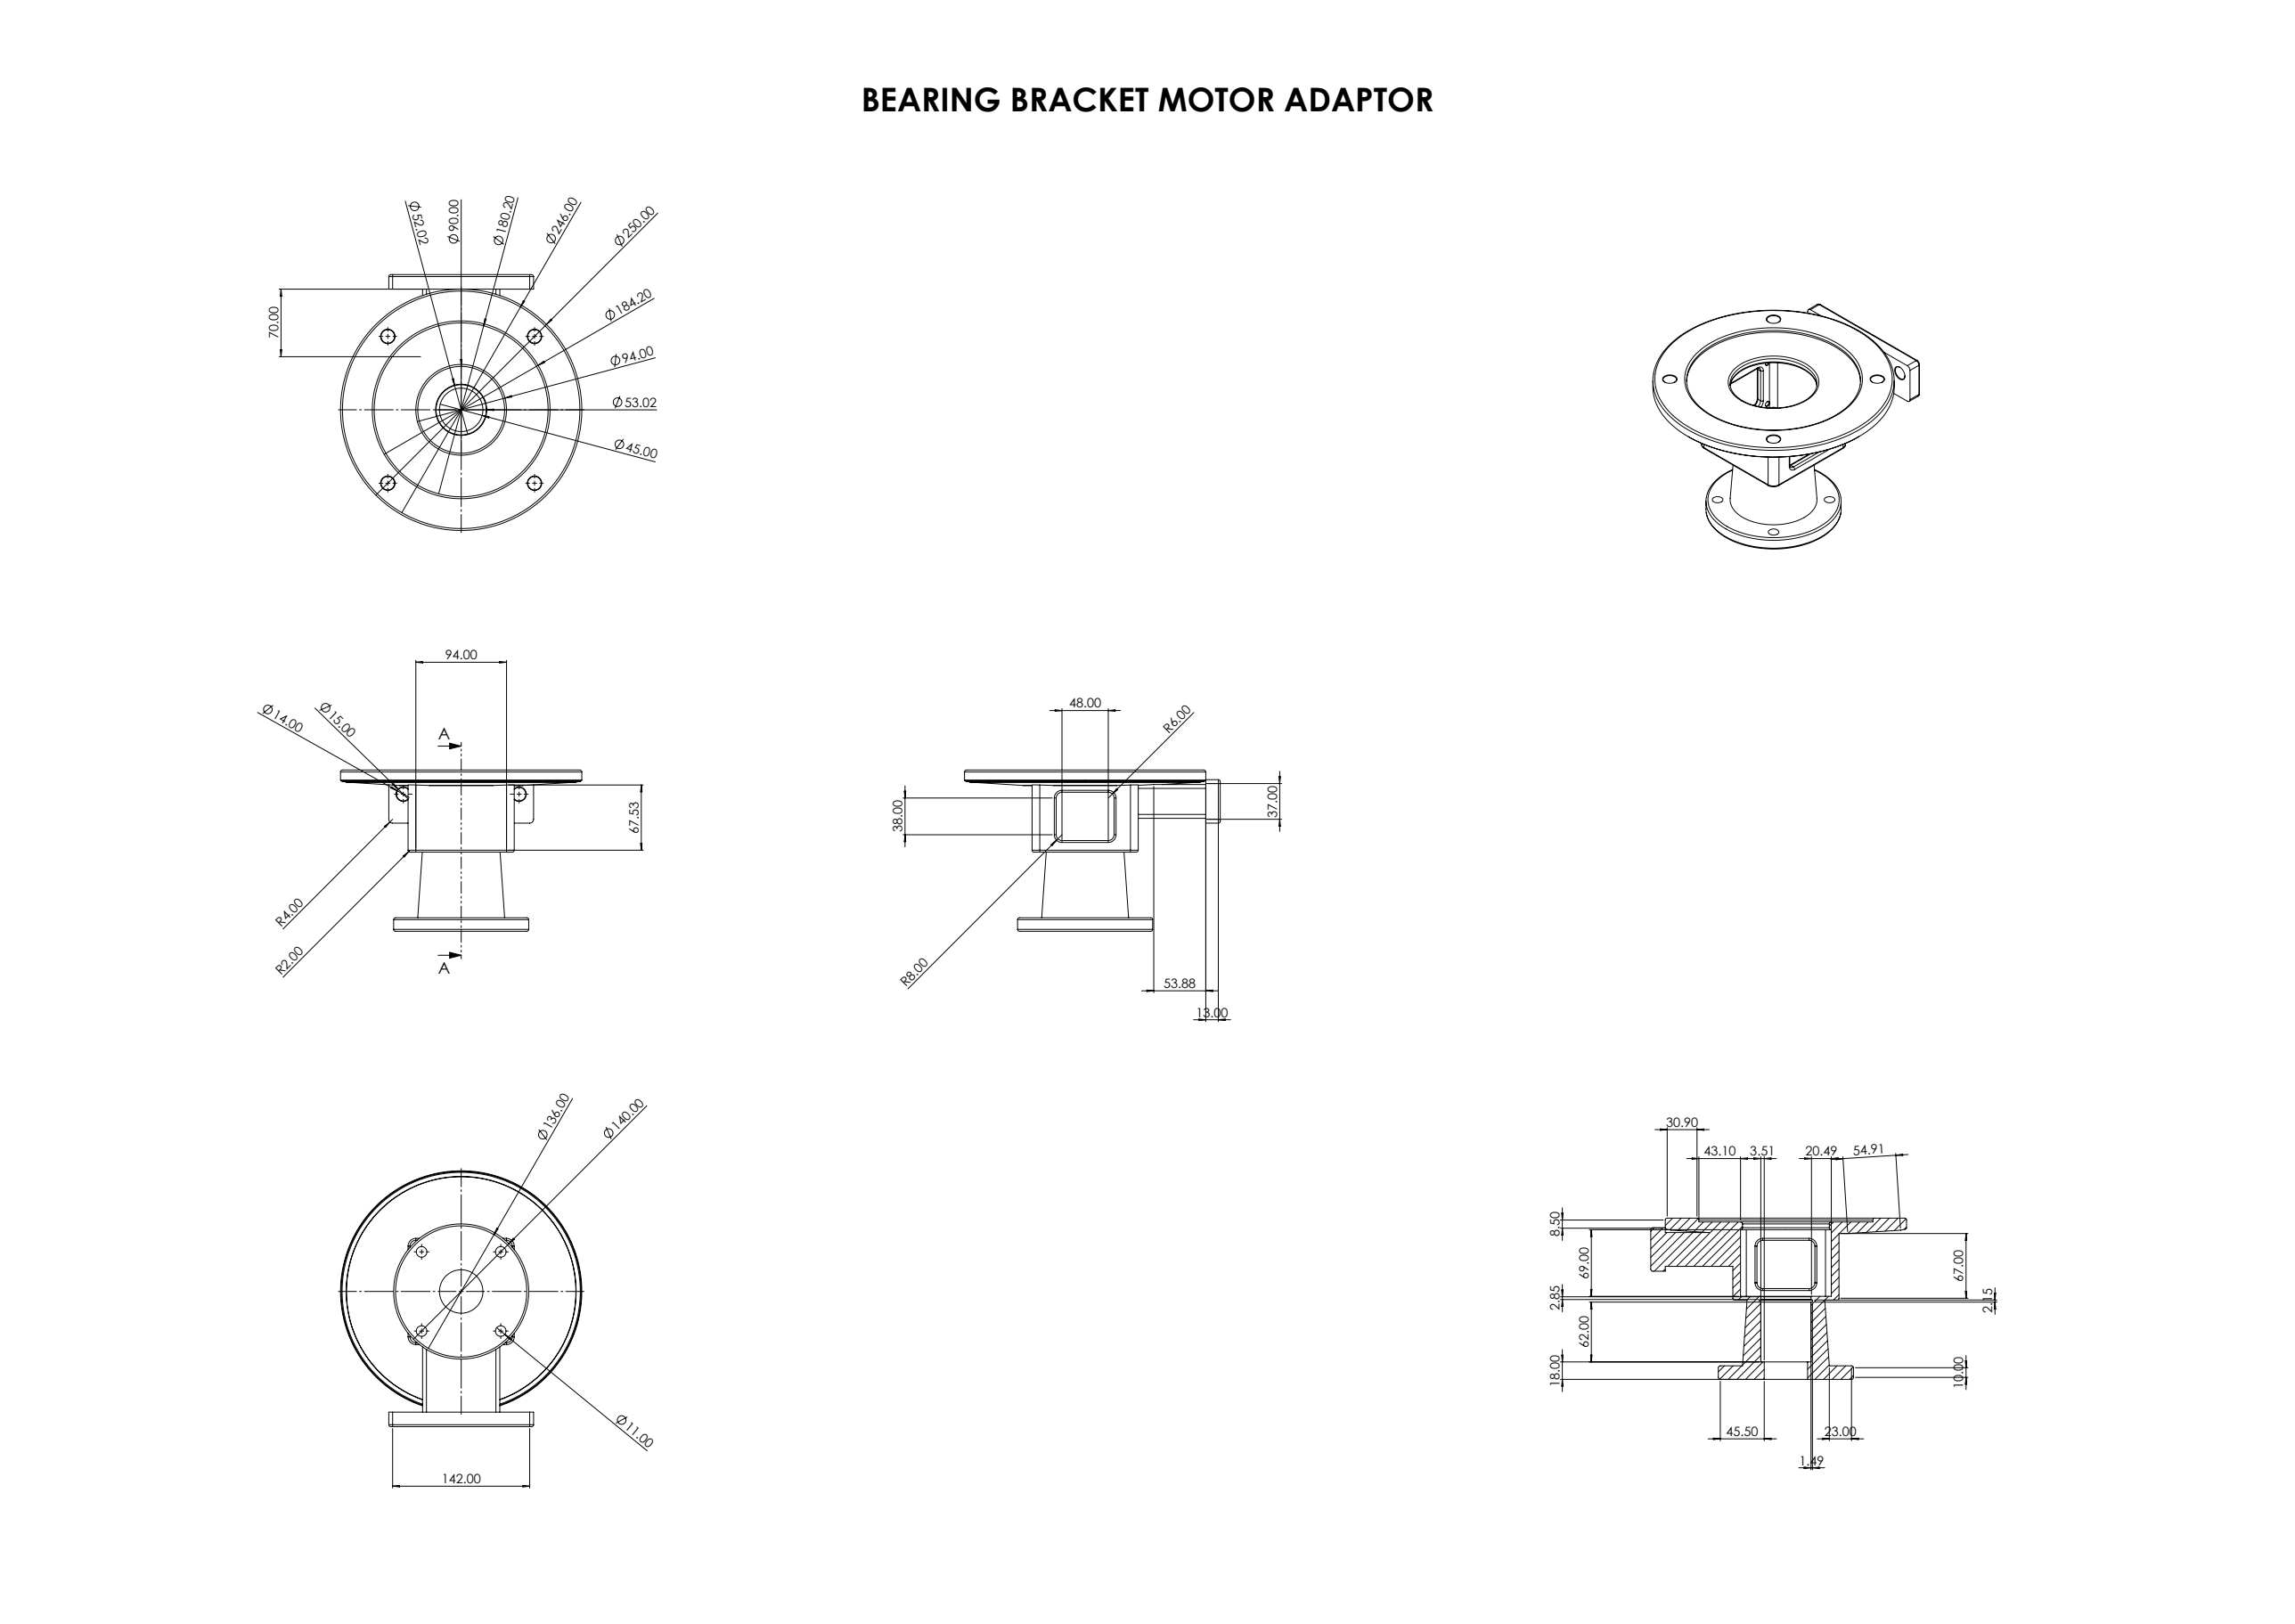
ISO-10303-21;
HEADER;
/* Generated by software containing ST-Developer
 * from STEP Tools, Inc. (www.steptools.com) 
 */

FILE_DESCRIPTION(
/* description */ (''),
/* implementation_level */ '2;1');

FILE_NAME(
/* name */ '03_Bearing_Bracket_Motor_Adaptor.step',
/* time_stamp */ '2026-10-26T04:15:57-07:00',
/* author */ (''),
/* organization */ (''),
/* preprocessor_version */ 'ST-DEVELOPER v20.2',
/* originating_system */ 'Autodesk Translation Framework v15.15.0.0',
/* authorisation */ '');

FILE_SCHEMA (('AUTOMOTIVE_DESIGN { 1 0 10303 214 3 1 1 }'));
ENDSEC;

DATA;
#10=MECHANICAL_DESIGN_GEOMETRIC_PRESENTATION_REPRESENTATION('',(#454),#55737);
#155=(
BOUNDED_CURVE()
B_SPLINE_CURVE(2,(#41789,#41790,#41791),.UNSPECIFIED.,.F.,.F.)
B_SPLINE_CURVE_WITH_KNOTS((3,3),(0.,1.18679419303782),.UNSPECIFIED.)
CURVE()
GEOMETRIC_REPRESENTATION_ITEM()
RATIONAL_B_SPLINE_CURVE((1.,1.03980835236638,1.06956749269866))
REPRESENTATION_ITEM('')
);
#156=(
BOUNDED_CURVE()
B_SPLINE_CURVE(2,(#41805,#41806,#41807),.UNSPECIFIED.,.F.,.F.)
B_SPLINE_CURVE_WITH_KNOTS((3,3),(8.21579802265979,9.40259221569659),
 .UNSPECIFIED.)
CURVE()
GEOMETRIC_REPRESENTATION_ITEM()
RATIONAL_B_SPLINE_CURVE((1.06956749269861,1.03980835236634,1.))
REPRESENTATION_ITEM('')
);
#157=(
BOUNDED_CURVE()
B_SPLINE_CURVE(2,(#41985,#41986,#41987),.UNSPECIFIED.,.F.,.F.)
B_SPLINE_CURVE_WITH_KNOTS((3,3),(0.,0.694054630120424),.UNSPECIFIED.)
CURVE()
GEOMETRIC_REPRESENTATION_ITEM()
RATIONAL_B_SPLINE_CURVE((1.,1.02328050763935,1.04312410261717))
REPRESENTATION_ITEM('')
);
#158=(
BOUNDED_CURVE()
B_SPLINE_CURVE(2,(#42011,#42012,#42013),.UNSPECIFIED.,.F.,.F.)
B_SPLINE_CURVE_WITH_KNOTS((3,3),(8.21579802265979,9.40259221569658),
 .UNSPECIFIED.)
CURVE()
GEOMETRIC_REPRESENTATION_ITEM()
RATIONAL_B_SPLINE_CURVE((1.06956749269861,1.03980835236634,1.))
REPRESENTATION_ITEM('')
);
#159=(
BOUNDED_CURVE()
B_SPLINE_CURVE(2,(#42017,#42018,#42019),.UNSPECIFIED.,.F.,.F.)
B_SPLINE_CURVE_WITH_KNOTS((3,3),(0.,1.18679419303782),.UNSPECIFIED.)
CURVE()
GEOMETRIC_REPRESENTATION_ITEM()
RATIONAL_B_SPLINE_CURVE((1.,1.03980835236638,1.06956749269866))
REPRESENTATION_ITEM('')
);
#160=(
BOUNDED_CURVE()
B_SPLINE_CURVE(2,(#42032,#42033,#42034),.UNSPECIFIED.,.F.,.F.)
B_SPLINE_CURVE_WITH_KNOTS((3,3),(8.21579802265979,9.40259221569659),
 .UNSPECIFIED.)
CURVE()
GEOMETRIC_REPRESENTATION_ITEM()
RATIONAL_B_SPLINE_CURVE((1.06956749269861,1.03980835236634,1.))
REPRESENTATION_ITEM('')
);
#161=(
BOUNDED_CURVE()
B_SPLINE_CURVE(2,(#42038,#42039,#42040),.UNSPECIFIED.,.F.,.F.)
B_SPLINE_CURVE_WITH_KNOTS((3,3),(0.,1.18679419303782),.UNSPECIFIED.)
CURVE()
GEOMETRIC_REPRESENTATION_ITEM()
RATIONAL_B_SPLINE_CURVE((1.,1.03980835236638,1.06956749269866))
REPRESENTATION_ITEM('')
);
#162=(
BOUNDED_CURVE()
B_SPLINE_CURVE(2,(#42053,#42054,#42055),.UNSPECIFIED.,.F.,.F.)
B_SPLINE_CURVE_WITH_KNOTS((3,3),(8.70853758557616,9.40259221569658),
 .UNSPECIFIED.)
CURVE()
GEOMETRIC_REPRESENTATION_ITEM()
RATIONAL_B_SPLINE_CURVE((1.04312410261717,1.02328050763935,1.))
REPRESENTATION_ITEM('')
);
#341=CONICAL_SURFACE('',#27990,26.26,0.785398163397439);
#342=CONICAL_SURFACE('',#28000,26.26,0.785398163397439);
#343=CONICAL_SURFACE('',#28004,7.25,0.785398163397439);
#344=CONICAL_SURFACE('',#28019,7.25,0.785398163397439);
#345=CONICAL_SURFACE('',#28023,2.8,0.785398163397448);
#346=CONICAL_SURFACE('',#28036,2.8,0.785398163397448);
#347=CONICAL_SURFACE('',#28043,2.8,0.785398163397448);
#348=CONICAL_SURFACE('',#28047,2.8,0.785398163397448);
#349=CONICAL_SURFACE('',#28052,2.8,0.785398163397448);
#350=CONICAL_SURFACE('',#28062,2.8,0.785398163397448);
#351=CONICAL_SURFACE('',#28063,2.8,0.785398163397448);
#352=CONICAL_SURFACE('',#28064,2.8,0.785398163397448);
#353=CONICAL_SURFACE('',#28065,7.25,0.785398163397439);
#354=CONICAL_SURFACE('',#28076,7.25,0.785398163397439);
#355=CONICAL_SURFACE('',#28080,7.25000000000001,0.785398163397448);
#356=CONICAL_SURFACE('',#28084,7.25,0.785398163397448);
#357=CONICAL_SURFACE('',#28088,7.25,0.785398163397439);
#358=CONICAL_SURFACE('',#28096,7.25,0.785398163397439);
#359=CONICAL_SURFACE('',#28122,121.5,1.37340076694501);
#360=CONICAL_SURFACE('',#28124,124.5,0.785398163397457);
#361=CONICAL_SURFACE('',#28129,91.5,1.50724565536944);
#362=CONICAL_SURFACE('',#28370,42.5,0.0693331336882086);
#414=SHAPE_REPRESENTATION_RELATIONSHIP('SRR','None',#55823,#434);
#434=ADVANCED_BREP_SHAPE_REPRESENTATION('',(#474),#55719);
#454=STYLED_ITEM('',(#55991),#474);
#474=MANIFOLD_SOLID_BREP('Body1',#27223);
#567=B_SPLINE_SURFACE_WITH_KNOTS('',3,3,((#41593,#41594,#41595,#41596),
(#41597,#41598,#41599,#41600),(#41601,#41602,#41603,#41604),(#41605,#41606,
#41607,#41608)),.UNSPECIFIED.,.F.,.F.,.F.,(4,4),(4,4),(0.,1.),(-3.32291242799128,
-2.9602728791883),.UNSPECIFIED.);
#568=B_SPLINE_SURFACE_WITH_KNOTS('',3,3,((#41671,#41672,#41673,#41674),
(#41675,#41676,#41677,#41678),(#41679,#41680,#41681,#41682),(#41683,#41684,
#41685,#41686)),.UNSPECIFIED.,.F.,.F.,.F.,(4,4),(4,4),(0.,1.),(-0.181319774401488,
0.181319774401493),.UNSPECIFIED.);
#569=B_SPLINE_SURFACE_WITH_KNOTS('',3,3,((#41713,#41714,#41715,#41716),
(#41717,#41718,#41719,#41720),(#41721,#41722,#41723,#41724),(#41725,#41726,
#41727,#41728)),.UNSPECIFIED.,.F.,.F.,.F.,(4,4),(4,4),(0.,1.),(-3.32291242799128,
-2.9602728791883),.UNSPECIFIED.);
#570=B_SPLINE_SURFACE_WITH_KNOTS('',3,3,((#41754,#41755,#41756,#41757),
(#41758,#41759,#41760,#41761),(#41762,#41763,#41764,#41765),(#41766,#41767,
#41768,#41769)),.UNSPECIFIED.,.F.,.F.,.F.,(4,4),(4,4),(0.,1.),(-6.46450508158109,
-6.10186553277809),.UNSPECIFIED.);
#600=(
BOUNDED_SURFACE()
B_SPLINE_SURFACE(2,2,((#42113,#42114,#42115),(#42116,#42117,#42118),(#42119,
#42120,#42121)),.UNSPECIFIED.,.F.,.F.,.F.)
B_SPLINE_SURFACE_WITH_KNOTS((3,3),(3,3),(-1.5707963267949,0.),(-3.14159265358979,
-1.5707963267949),.UNSPECIFIED.)
GEOMETRIC_REPRESENTATION_ITEM()
RATIONAL_B_SPLINE_SURFACE(((1.,0.707106781186548,1.),(0.707106781186538,
0.499999999999993,0.707106781186538),(1.,0.707106781186548,1.)))
REPRESENTATION_ITEM('')
SURFACE()
);
#601=(
BOUNDED_SURFACE()
B_SPLINE_SURFACE(2,2,((#42129,#42130,#42131),(#42132,#42133,#42134),(#42135,
#42136,#42137)),.UNSPECIFIED.,.F.,.F.,.F.)
B_SPLINE_SURFACE_WITH_KNOTS((3,3),(3,3),(-1.57079632679491,0.),(-1.5707963267949,
0.),.UNSPECIFIED.)
GEOMETRIC_REPRESENTATION_ITEM()
RATIONAL_B_SPLINE_SURFACE(((1.,0.707106781186546,1.),(0.707106781186548,
0.499999999999999,0.707106781186548),(1.,0.707106781186546,1.)))
REPRESENTATION_ITEM('')
SURFACE()
);
#602=(
BOUNDED_SURFACE()
B_SPLINE_SURFACE(2,2,((#42145,#42146,#42147),(#42148,#42149,#42150),(#42151,
#42152,#42153)),.UNSPECIFIED.,.F.,.F.,.F.)
B_SPLINE_SURFACE_WITH_KNOTS((3,3),(3,3),(-1.5707963267949,0.),(0.,1.5707963267949),
 .UNSPECIFIED.)
GEOMETRIC_REPRESENTATION_ITEM()
RATIONAL_B_SPLINE_SURFACE(((1.,0.707106781186548,1.),(0.707106781186538,
0.499999999999993,0.707106781186538),(1.,0.707106781186548,1.)))
REPRESENTATION_ITEM('')
SURFACE()
);
#603=(
BOUNDED_SURFACE()
B_SPLINE_SURFACE(2,2,((#42161,#42162,#42163),(#42164,#42165,#42166),(#42167,
#42168,#42169)),.UNSPECIFIED.,.F.,.F.,.F.)
B_SPLINE_SURFACE_WITH_KNOTS((3,3),(3,3),(-1.57079632679491,0.),(1.57079632679489,
3.14159265358979),.UNSPECIFIED.)
GEOMETRIC_REPRESENTATION_ITEM()
RATIONAL_B_SPLINE_SURFACE(((1.,0.707106781186546,1.),(0.707106781186548,
0.499999999999999,0.707106781186548),(1.,0.707106781186546,1.)))
REPRESENTATION_ITEM('')
SURFACE()
);
#647=FACE_BOUND('',#8787,.T.);
#648=FACE_BOUND('',#8790,.T.);
#649=FACE_BOUND('',#8793,.T.);
#650=FACE_BOUND('',#8794,.T.);
#651=FACE_BOUND('',#8795,.T.);
#652=FACE_BOUND('',#8802,.T.);
#653=FACE_BOUND('',#8816,.T.);
#654=FACE_BOUND('',#8817,.T.);
#655=FACE_BOUND('',#8818,.T.);
#656=FACE_BOUND('',#8819,.T.);
#657=FACE_BOUND('',#8820,.T.);
#658=FACE_BOUND('',#8826,.T.);
#659=FACE_BOUND('',#8827,.T.);
#660=FACE_BOUND('',#8828,.T.);
#661=FACE_BOUND('',#8829,.T.);
#662=FACE_BOUND('',#8830,.T.);
#663=FACE_BOUND('',#8840,.T.);
#664=FACE_BOUND('',#8841,.T.);
#665=FACE_BOUND('',#8846,.T.);
#666=FACE_BOUND('',#8847,.T.);
#667=FACE_BOUND('',#8848,.T.);
#668=FACE_BOUND('',#8849,.T.);
#669=FACE_BOUND('',#8850,.T.);
#670=FACE_BOUND('',#8853,.T.);
#671=FACE_BOUND('',#8854,.T.);
#672=FACE_BOUND('',#8855,.T.);
#673=FACE_BOUND('',#8856,.T.);
#674=FACE_BOUND('',#8857,.T.);
#675=FACE_BOUND('',#8893,.T.);
#676=FACE_BOUND('',#8907,.T.);
#677=FACE_BOUND('',#8920,.T.);
#678=FACE_BOUND('',#8933,.T.);
#679=FACE_BOUND('',#8968,.T.);
#680=FACE_BOUND('',#8971,.T.);
#883=PLANE('',#27995);
#884=PLANE('',#28002);
#885=PLANE('',#28007);
#886=PLANE('',#28026);
#887=PLANE('',#28054);
#888=PLANE('',#28068);
#889=PLANE('',#28090);
#890=PLANE('',#28103);
#891=PLANE('',#28112);
#892=PLANE('',#28137);
#893=PLANE('',#28140);
#894=PLANE('',#28143);
#895=PLANE('',#28161);
#896=PLANE('',#28163);
#897=PLANE('',#28175);
#898=PLANE('',#28177);
#899=PLANE('',#28179);
#900=PLANE('',#28180);
#901=PLANE('',#28193);
#902=PLANE('',#28220);
#903=PLANE('',#28223);
#904=PLANE('',#28224);
#905=PLANE('',#28248);
#906=PLANE('',#28250);
#907=PLANE('',#28276);
#908=PLANE('',#28282);
#909=PLANE('',#28306);
#910=PLANE('',#28309);
#911=PLANE('',#28329);
#912=PLANE('',#28331);
#913=PLANE('',#28332);
#914=PLANE('',#28333);
#915=PLANE('',#28334);
#916=PLANE('',#28339);
#917=PLANE('',#28340);
#918=PLANE('',#28341);
#919=PLANE('',#28345);
#920=PLANE('',#28350);
#921=PLANE('',#28352);
#922=PLANE('',#28354);
#923=PLANE('',#28356);
#924=PLANE('',#28358);
#925=PLANE('',#28360);
#926=PLANE('',#28362);
#927=PLANE('',#28364);
#928=PLANE('',#28366);
#2176=LINE('',#41497,#4547);
#2177=LINE('',#41502,#4548);
#2178=LINE('',#41508,#4549);
#2179=LINE('',#41512,#4550);
#2180=LINE('',#41516,#4551);
#2181=LINE('',#41519,#4552);
#2182=LINE('',#41522,#4553);
#2183=LINE('',#41531,#4554);
#2184=LINE('',#41538,#4555);
#2185=LINE('',#41542,#4556);
#2186=LINE('',#41546,#4557);
#2187=LINE('',#41548,#4558);
#2188=LINE('',#41550,#4559);
#2189=LINE('',#41553,#4560);
#2190=LINE('',#41558,#4561);
#2191=LINE('',#41562,#4562);
#2192=LINE('',#41566,#4563);
#2193=LINE('',#41570,#4564);
#2194=LINE('',#41574,#4565);
#2195=LINE('',#41578,#4566);
#2196=LINE('',#41582,#4567);
#2197=LINE('',#41587,#4568);
#2198=LINE('',#41591,#4569);
#2199=LINE('',#41624,#4570);
#2200=LINE('',#41627,#4571);
#2201=LINE('',#41629,#4572);
#2202=LINE('',#41633,#4573);
#2203=LINE('',#41637,#4574);
#2204=LINE('',#41639,#4575);
#2205=LINE('',#41641,#4576);
#2206=LINE('',#41642,#4577);
#2207=LINE('',#41645,#4578);
#2208=LINE('',#41649,#4579);
#2209=LINE('',#41653,#4580);
#2210=LINE('',#41657,#4581);
#2211=LINE('',#41662,#4582);
#2212=LINE('',#41665,#4583);
#2213=LINE('',#41670,#4584);
#2214=LINE('',#41697,#4585);
#2215=LINE('',#41706,#4586);
#2216=LINE('',#41709,#4587);
#2217=LINE('',#41712,#4588);
#2218=LINE('',#41745,#4589);
#2219=LINE('',#41748,#4590);
#2220=LINE('',#41753,#4591);
#2221=LINE('',#41777,#4592);
#2222=LINE('',#41781,#4593);
#2223=LINE('',#41785,#4594);
#2224=LINE('',#41787,#4595);
#2225=LINE('',#41798,#4596);
#2226=LINE('',#41808,#4597);
#2227=LINE('',#41815,#4598);
#2228=LINE('',#41819,#4599);
#2229=LINE('',#41823,#4600);
#2230=LINE('',#41827,#4601);
#2231=LINE('',#41832,#4602);
#2232=LINE('',#41834,#4603);
#2233=LINE('',#41836,#4604);
#2234=LINE('',#41841,#4605);
#2235=LINE('',#41857,#4606);
#2236=LINE('',#41860,#4607);
#2237=LINE('',#41865,#4608);
#2238=LINE('',#41868,#4609);
#2239=LINE('',#41873,#4610);
#2240=LINE('',#41876,#4611);
#2241=LINE('',#41881,#4612);
#2242=LINE('',#41885,#4613);
#2243=LINE('',#41889,#4614);
#2244=LINE('',#41893,#4615);
#2245=LINE('',#41897,#4616);
#2246=LINE('',#41901,#4617);
#2247=LINE('',#41906,#4618);
#2248=LINE('',#41915,#4619);
#2249=LINE('',#41951,#4620);
#2250=LINE('',#41955,#4621);
#2251=LINE('',#41962,#4622);
#2252=LINE('',#42089,#4623);
#2253=LINE('',#42103,#4624);
#2254=LINE('',#42112,#4625);
#2255=LINE('',#42128,#4626);
#2256=LINE('',#42144,#4627);
#2257=LINE('',#42160,#4628);
#2258=LINE('',#42172,#4629);
#2259=LINE('',#42173,#4630);
#2260=LINE('',#42175,#4631);
#2261=LINE('',#42177,#4632);
#2262=LINE('',#42179,#4633);
#2263=LINE('',#42185,#4634);
#2264=LINE('',#42186,#4635);
#2265=LINE('',#42200,#4636);
#2266=LINE('',#42203,#4637);
#2267=LINE('',#42206,#4638);
#2268=LINE('',#42209,#4639);
#2269=LINE('',#42211,#4640);
#2270=LINE('',#42214,#4641);
#2271=LINE('',#42219,#4642);
#2272=LINE('',#42229,#4643);
#2273=LINE('',#42240,#4644);
#2274=LINE('',#42243,#4645);
#2275=LINE('',#42254,#4646);
#2276=LINE('',#42255,#4647);
#2277=LINE('',#42266,#4648);
#2278=LINE('',#42267,#4649);
#2279=LINE('',#42278,#4650);
#2280=LINE('',#42279,#4651);
#2281=LINE('',#42285,#4652);
#2282=LINE('',#42288,#4653);
#2283=LINE('',#42291,#4654);
#2284=LINE('',#42292,#4655);
#2285=LINE('',#42295,#4656);
#2286=LINE('',#42299,#4657);
#2287=LINE('',#42300,#4658);
#2288=LINE('',#42304,#4659);
#2289=LINE('',#42305,#4660);
#2290=LINE('',#42306,#4661);
#2291=LINE('',#42312,#4662);
#2292=LINE('',#42323,#4663);
#2293=LINE('',#42324,#4664);
#2294=LINE('',#42334,#4665);
#2295=LINE('',#42335,#4666);
#2296=LINE('',#42343,#4667);
#2297=LINE('',#42347,#4668);
#2298=LINE('',#42348,#4669);
#2299=LINE('',#42350,#4670);
#2300=LINE('',#42353,#4671);
#2301=LINE('',#42354,#4672);
#2302=LINE('',#42360,#4673);
#2303=LINE('',#42371,#4674);
#2304=LINE('',#42372,#4675);
#2305=LINE('',#42381,#4676);
#2306=LINE('',#42392,#4677);
#2307=LINE('',#42393,#4678);
#2308=LINE('',#42398,#4679);
#2309=LINE('',#42400,#4680);
#2310=LINE('',#42404,#4681);
#2311=LINE('',#42408,#4682);
#2312=LINE('',#42412,#4683);
#2313=LINE('',#42422,#4684);
#2314=LINE('',#42431,#4685);
#2315=LINE('',#42439,#4686);
#2316=LINE('',#42447,#4687);
#2317=LINE('',#42452,#4688);
#2318=LINE('',#42455,#4689);
#2319=LINE('',#42458,#4690);
#2320=LINE('',#42459,#4691);
#2321=LINE('',#42462,#4692);
#2322=LINE('',#42466,#4693);
#2323=LINE('',#42467,#4694);
#2324=LINE('',#42478,#4695);
#2325=LINE('',#42485,#4696);
#2326=LINE('',#42492,#4697);
#2327=LINE('',#42493,#4698);
#2328=LINE('',#42495,#4699);
#2329=LINE('',#42502,#4700);
#2330=LINE('',#42504,#4701);
#2331=LINE('',#42506,#4702);
#2332=LINE('',#42508,#4703);
#2333=LINE('',#42517,#4704);
#2334=LINE('',#42524,#4705);
#2335=LINE('',#42526,#4706);
#2336=LINE('',#42528,#4707);
#2337=LINE('',#42531,#4708);
#2338=LINE('',#42534,#4709);
#2339=LINE('',#42536,#4710);
#2340=LINE('',#42538,#4711);
#2341=LINE('',#42541,#4712);
#2342=LINE('',#42542,#4713);
#2343=LINE('',#42544,#4714);
#2344=LINE('',#42546,#4715);
#2345=LINE('',#42548,#4716);
#2346=LINE('',#42550,#4717);
#2347=LINE('',#42552,#4718);
#2348=LINE('',#42554,#4719);
#2349=LINE('',#42557,#4720);
#2350=LINE('',#42558,#4721);
#2351=LINE('',#42562,#4722);
#2352=LINE('',#42564,#4723);
#4547=VECTOR('',#31454,26.26);
#4548=VECTOR('',#31461,26.01);
#4549=VECTOR('',#31466,10.);
#4550=VECTOR('',#31469,10.);
#4551=VECTOR('',#31472,10.);
#4552=VECTOR('',#31475,10.);
#4553=VECTOR('',#31478,26.26);
#4554=VECTOR('',#31489,7.25);
#4555=VECTOR('',#31496,10.);
#4556=VECTOR('',#31499,10.);
#4557=VECTOR('',#31502,10.);
#4558=VECTOR('',#31503,10.);
#4559=VECTOR('',#31504,10.);
#4560=VECTOR('',#31507,10.);
#4561=VECTOR('',#31510,10.);
#4562=VECTOR('',#31513,10.);
#4563=VECTOR('',#31516,10.);
#4564=VECTOR('',#31519,10.);
#4565=VECTOR('',#31524,7.);
#4566=VECTOR('',#31529,7.25);
#4567=VECTOR('',#31534,7.);
#4568=VECTOR('',#31539,10.);
#4569=VECTOR('',#31542,10.);
#4570=VECTOR('',#31547,10.);
#4571=VECTOR('',#31550,10.);
#4572=VECTOR('',#31551,10.);
#4573=VECTOR('',#31554,10.);
#4574=VECTOR('',#31557,10.);
#4575=VECTOR('',#31558,10.);
#4576=VECTOR('',#31559,10.);
#4577=VECTOR('',#31560,10.);
#4578=VECTOR('',#31561,10.);
#4579=VECTOR('',#31564,10.);
#4580=VECTOR('',#31567,10.);
#4581=VECTOR('',#31570,10.);
#4582=VECTOR('',#31577,2.55);
#4583=VECTOR('',#31580,10.);
#4584=VECTOR('',#31585,10.);
#4585=VECTOR('',#31588,10.);
#4586=VECTOR('',#31595,2.55);
#4587=VECTOR('',#31598,10.);
#4588=VECTOR('',#31601,10.);
#4589=VECTOR('',#31606,2.55);
#4590=VECTOR('',#31609,10.);
#4591=VECTOR('',#31614,10.);
#4592=VECTOR('',#31619,2.55);
#4593=VECTOR('',#31624,2.8);
#4594=VECTOR('',#31627,10.);
#4595=VECTOR('',#31628,10.);
#4596=VECTOR('',#31629,10.);
#4597=VECTOR('',#31630,10.);
#4598=VECTOR('',#31635,10.);
#4599=VECTOR('',#31638,10.);
#4600=VECTOR('',#31641,10.);
#4601=VECTOR('',#31644,10.);
#4602=VECTOR('',#31651,2.8);
#4603=VECTOR('',#31654,2.8);
#4604=VECTOR('',#31657,2.8);
#4605=VECTOR('',#31662,7.25);
#4606=VECTOR('',#31681,7.);
#4607=VECTOR('',#31684,7.25);
#4608=VECTOR('',#31691,7.);
#4609=VECTOR('',#31694,7.25000000000001);
#4610=VECTOR('',#31701,7.);
#4611=VECTOR('',#31704,7.25);
#4612=VECTOR('',#31711,6.99999999999999);
#4613=VECTOR('',#31716,7.25);
#4614=VECTOR('',#31719,10.);
#4615=VECTOR('',#31722,10.);
#4616=VECTOR('',#31725,10.);
#4617=VECTOR('',#31728,10.);
#4618=VECTOR('',#31735,7.25);
#4619=VECTOR('',#31746,70.);
#4620=VECTOR('',#31789,121.5);
#4621=VECTOR('',#31796,124.5);
#4622=VECTOR('',#31805,91.5);
#4623=VECTOR('',#31822,10.);
#4624=VECTOR('',#31829,10.);
#4625=VECTOR('',#31842,10.);
#4626=VECTOR('',#31851,10.);
#4627=VECTOR('',#31860,10.);
#4628=VECTOR('',#31869,10.);
#4629=VECTOR('',#31874,10.);
#4630=VECTOR('',#31875,10.);
#4631=VECTOR('',#31878,10.);
#4632=VECTOR('',#31881,10.);
#4633=VECTOR('',#31884,10.);
#4634=VECTOR('',#31893,125.);
#4635=VECTOR('',#31894,10.);
#4636=VECTOR('',#31911,10.);
#4637=VECTOR('',#31914,10.);
#4638=VECTOR('',#31917,10.);
#4639=VECTOR('',#31920,10.);
#4640=VECTOR('',#31923,10.);
#4641=VECTOR('',#31926,10.);
#4642=VECTOR('',#31933,45.);
#4643=VECTOR('',#31946,90.1);
#4644=VECTOR('',#31959,10.);
#4645=VECTOR('',#31962,10.);
#4646=VECTOR('',#31975,10.);
#4647=VECTOR('',#31976,10.);
#4648=VECTOR('',#31989,10.);
#4649=VECTOR('',#31990,10.);
#4650=VECTOR('',#32003,10.);
#4651=VECTOR('',#32004,10.);
#4652=VECTOR('',#32013,10.);
#4653=VECTOR('',#32016,10.);
#4654=VECTOR('',#32019,10.);
#4655=VECTOR('',#32020,10.);
#4656=VECTOR('',#32023,10.);
#4657=VECTOR('',#32028,10.);
#4658=VECTOR('',#32029,10.);
#4659=VECTOR('',#32032,10.);
#4660=VECTOR('',#32033,10.);
#4661=VECTOR('',#32034,10.);
#4662=VECTOR('',#32041,10.);
#4663=VECTOR('',#32054,10.);
#4664=VECTOR('',#32055,10.);
#4665=VECTOR('',#32068,10.);
#4666=VECTOR('',#32069,10.);
#4667=VECTOR('',#32080,10.);
#4668=VECTOR('',#32087,10.);
#4669=VECTOR('',#32088,10.);
#4670=VECTOR('',#32091,10.);
#4671=VECTOR('',#32096,10.);
#4672=VECTOR('',#32097,10.);
#4673=VECTOR('',#32104,10.);
#4674=VECTOR('',#32117,10.);
#4675=VECTOR('',#32118,10.);
#4676=VECTOR('',#32131,10.);
#4677=VECTOR('',#32144,10.);
#4678=VECTOR('',#32145,10.);
#4679=VECTOR('',#32154,10.);
#4680=VECTOR('',#32157,10.);
#4681=VECTOR('',#32160,10.);
#4682=VECTOR('',#32163,10.);
#4683=VECTOR('',#32166,10.);
#4684=VECTOR('',#32179,10.);
#4685=VECTOR('',#32192,10.);
#4686=VECTOR('',#32203,10.);
#4687=VECTOR('',#32214,10.);
#4688=VECTOR('',#32221,10.);
#4689=VECTOR('',#32224,10.);
#4690=VECTOR('',#32227,10.);
#4691=VECTOR('',#32228,10.);
#4692=VECTOR('',#32231,10.);
#4693=VECTOR('',#32236,10.);
#4694=VECTOR('',#32237,10.);
#4695=VECTOR('',#32254,10.);
#4696=VECTOR('',#32265,10.);
#4697=VECTOR('',#32278,10.);
#4698=VECTOR('',#32279,10.);
#4699=VECTOR('',#32282,10.);
#4700=VECTOR('',#32295,5.5);
#4701=VECTOR('',#32298,5.5);
#4702=VECTOR('',#32301,5.5);
#4703=VECTOR('',#32304,5.5);
#4704=VECTOR('',#32317,27.5);
#4705=VECTOR('',#32326,26.01);
#4706=VECTOR('',#32329,10.);
#4707=VECTOR('',#32332,10.);
#4708=VECTOR('',#32337,10.);
#4709=VECTOR('',#32342,10.);
#4710=VECTOR('',#32345,10.);
#4711=VECTOR('',#32348,10.);
#4712=VECTOR('',#32353,10.);
#4713=VECTOR('',#32354,10.);
#4714=VECTOR('',#32357,10.);
#4715=VECTOR('',#32360,10.);
#4716=VECTOR('',#32363,10.);
#4717=VECTOR('',#32366,10.);
#4718=VECTOR('',#32369,10.);
#4719=VECTOR('',#32372,10.);
#4720=VECTOR('',#32377,10.);
#4721=VECTOR('',#32378,10.);
#4722=VECTOR('',#32385,22.5);
#4723=VECTOR('',#32388,42.5);
#6602=CYLINDRICAL_SURFACE('',#27993,26.01);
#6603=CYLINDRICAL_SURFACE('',#28017,7.);
#6604=CYLINDRICAL_SURFACE('',#28021,7.);
#6605=CYLINDRICAL_SURFACE('',#28034,2.55);
#6606=CYLINDRICAL_SURFACE('',#28039,6.00000000000002);
#6607=CYLINDRICAL_SURFACE('',#28041,2.55);
#6608=CYLINDRICAL_SURFACE('',#28045,2.55);
#6609=CYLINDRICAL_SURFACE('',#28050,2.55);
#6610=CYLINDRICAL_SURFACE('',#28074,7.);
#6611=CYLINDRICAL_SURFACE('',#28078,7.);
#6612=CYLINDRICAL_SURFACE('',#28082,7.);
#6613=CYLINDRICAL_SURFACE('',#28086,6.99999999999999);
#6614=CYLINDRICAL_SURFACE('',#28101,70.);
#6615=CYLINDRICAL_SURFACE('',#28144,2.);
#6616=CYLINDRICAL_SURFACE('',#28149,2.);
#6617=CYLINDRICAL_SURFACE('',#28153,2.);
#6618=CYLINDRICAL_SURFACE('',#28157,2.);
#6619=CYLINDRICAL_SURFACE('',#28160,4.);
#6620=CYLINDRICAL_SURFACE('',#28162,3.99999999999999);
#6621=CYLINDRICAL_SURFACE('',#28167,125.);
#6622=CYLINDRICAL_SURFACE('',#28182,45.);
#6623=CYLINDRICAL_SURFACE('',#28188,90.1);
#6624=CYLINDRICAL_SURFACE('',#28194,2.);
#6625=CYLINDRICAL_SURFACE('',#28201,2.);
#6626=CYLINDRICAL_SURFACE('',#28207,2.);
#6627=CYLINDRICAL_SURFACE('',#28213,2.);
#6628=CYLINDRICAL_SURFACE('',#28218,5.99999999999999);
#6629=CYLINDRICAL_SURFACE('',#28221,5.99999999999998);
#6630=CYLINDRICAL_SURFACE('',#28225,2.);
#6631=CYLINDRICAL_SURFACE('',#28232,2.);
#6632=CYLINDRICAL_SURFACE('',#28238,2.);
#6633=CYLINDRICAL_SURFACE('',#28243,2.);
#6634=CYLINDRICAL_SURFACE('',#28247,6.00000000000001);
#6635=CYLINDRICAL_SURFACE('',#28249,6.00000000000001);
#6636=CYLINDRICAL_SURFACE('',#28251,2.);
#6637=CYLINDRICAL_SURFACE('',#28258,2.);
#6638=CYLINDRICAL_SURFACE('',#28264,2.);
#6639=CYLINDRICAL_SURFACE('',#28270,2.);
#6640=CYLINDRICAL_SURFACE('',#28275,8.);
#6641=CYLINDRICAL_SURFACE('',#28281,8.);
#6642=CYLINDRICAL_SURFACE('',#28284,2.);
#6643=CYLINDRICAL_SURFACE('',#28290,2.);
#6644=CYLINDRICAL_SURFACE('',#28295,2.);
#6645=CYLINDRICAL_SURFACE('',#28300,2.);
#6646=CYLINDRICAL_SURFACE('',#28304,6.00000000000001);
#6647=CYLINDRICAL_SURFACE('',#28307,5.99999999999998);
#6648=CYLINDRICAL_SURFACE('',#28310,2.);
#6649=CYLINDRICAL_SURFACE('',#28316,2.);
#6650=CYLINDRICAL_SURFACE('',#28321,2.);
#6651=CYLINDRICAL_SURFACE('',#28325,2.);
#6652=CYLINDRICAL_SURFACE('',#28328,6.00000000000001);
#6653=CYLINDRICAL_SURFACE('',#28330,5.99999999999999);
#6654=CYLINDRICAL_SURFACE('',#28335,5.5);
#6655=CYLINDRICAL_SURFACE('',#28336,5.5);
#6656=CYLINDRICAL_SURFACE('',#28337,5.5);
#6657=CYLINDRICAL_SURFACE('',#28338,5.5);
#6658=CYLINDRICAL_SURFACE('',#28344,27.5);
#6659=CYLINDRICAL_SURFACE('',#28348,26.01);
#6660=CYLINDRICAL_SURFACE('',#28349,6.00000000000002);
#6661=CYLINDRICAL_SURFACE('',#28351,6.00000000000002);
#6662=CYLINDRICAL_SURFACE('',#28353,6.00000000000002);
#6663=CYLINDRICAL_SURFACE('',#28355,3.99999999999999);
#6664=CYLINDRICAL_SURFACE('',#28357,4.);
#6665=CYLINDRICAL_SURFACE('',#28359,3.99999999999998);
#6666=CYLINDRICAL_SURFACE('',#28361,3.99999999999999);
#6667=CYLINDRICAL_SURFACE('',#28363,3.99999999999998);
#6668=CYLINDRICAL_SURFACE('',#28365,3.99999999999999);
#6669=CYLINDRICAL_SURFACE('',#28367,8.);
#6670=CYLINDRICAL_SURFACE('',#28368,8.);
#6671=CYLINDRICAL_SURFACE('',#28369,22.5);
#7172=FACE_OUTER_BOUND('',#8784,.T.);
#7173=FACE_OUTER_BOUND('',#8785,.T.);
#7174=FACE_OUTER_BOUND('',#8786,.T.);
#7175=FACE_OUTER_BOUND('',#8788,.T.);
#7176=FACE_OUTER_BOUND('',#8789,.T.);
#7177=FACE_OUTER_BOUND('',#8791,.T.);
#7178=FACE_OUTER_BOUND('',#8792,.T.);
#7179=FACE_OUTER_BOUND('',#8796,.T.);
#7180=FACE_OUTER_BOUND('',#8797,.T.);
#7181=FACE_OUTER_BOUND('',#8798,.T.);
#7182=FACE_OUTER_BOUND('',#8799,.T.);
#7183=FACE_OUTER_BOUND('',#8800,.T.);
#7184=FACE_OUTER_BOUND('',#8801,.T.);
#7185=FACE_OUTER_BOUND('',#8803,.T.);
#7186=FACE_OUTER_BOUND('',#8804,.T.);
#7187=FACE_OUTER_BOUND('',#8805,.T.);
#7188=FACE_OUTER_BOUND('',#8806,.T.);
#7189=FACE_OUTER_BOUND('',#8807,.T.);
#7190=FACE_OUTER_BOUND('',#8808,.T.);
#7191=FACE_OUTER_BOUND('',#8809,.T.);
#7192=FACE_OUTER_BOUND('',#8810,.T.);
#7193=FACE_OUTER_BOUND('',#8811,.T.);
#7194=FACE_OUTER_BOUND('',#8812,.T.);
#7195=FACE_OUTER_BOUND('',#8813,.T.);
#7196=FACE_OUTER_BOUND('',#8814,.T.);
#7197=FACE_OUTER_BOUND('',#8815,.T.);
#7198=FACE_OUTER_BOUND('',#8821,.T.);
#7199=FACE_OUTER_BOUND('',#8822,.T.);
#7200=FACE_OUTER_BOUND('',#8823,.T.);
#7201=FACE_OUTER_BOUND('',#8824,.T.);
#7202=FACE_OUTER_BOUND('',#8825,.T.);
#7203=FACE_OUTER_BOUND('',#8831,.T.);
#7204=FACE_OUTER_BOUND('',#8832,.T.);
#7205=FACE_OUTER_BOUND('',#8833,.T.);
#7206=FACE_OUTER_BOUND('',#8834,.T.);
#7207=FACE_OUTER_BOUND('',#8835,.T.);
#7208=FACE_OUTER_BOUND('',#8836,.T.);
#7209=FACE_OUTER_BOUND('',#8837,.T.);
#7210=FACE_OUTER_BOUND('',#8838,.T.);
#7211=FACE_OUTER_BOUND('',#8839,.T.);
#7212=FACE_OUTER_BOUND('',#8842,.T.);
#7213=FACE_OUTER_BOUND('',#8843,.T.);
#7214=FACE_OUTER_BOUND('',#8844,.T.);
#7215=FACE_OUTER_BOUND('',#8845,.T.);
#7216=FACE_OUTER_BOUND('',#8851,.T.);
#7217=FACE_OUTER_BOUND('',#8852,.T.);
#7218=FACE_OUTER_BOUND('',#8858,.T.);
#7219=FACE_OUTER_BOUND('',#8859,.T.);
#7220=FACE_OUTER_BOUND('',#8860,.T.);
#7221=FACE_OUTER_BOUND('',#8861,.T.);
#7222=FACE_OUTER_BOUND('',#8862,.T.);
#7223=FACE_OUTER_BOUND('',#8863,.T.);
#7224=FACE_OUTER_BOUND('',#8864,.T.);
#7225=FACE_OUTER_BOUND('',#8865,.T.);
#7226=FACE_OUTER_BOUND('',#8866,.T.);
#7227=FACE_OUTER_BOUND('',#8867,.T.);
#7228=FACE_OUTER_BOUND('',#8868,.T.);
#7229=FACE_OUTER_BOUND('',#8869,.T.);
#7230=FACE_OUTER_BOUND('',#8870,.T.);
#7231=FACE_OUTER_BOUND('',#8871,.T.);
#7232=FACE_OUTER_BOUND('',#8872,.T.);
#7233=FACE_OUTER_BOUND('',#8873,.T.);
#7234=FACE_OUTER_BOUND('',#8874,.T.);
#7235=FACE_OUTER_BOUND('',#8875,.T.);
#7236=FACE_OUTER_BOUND('',#8876,.T.);
#7237=FACE_OUTER_BOUND('',#8877,.T.);
#7238=FACE_OUTER_BOUND('',#8878,.T.);
#7239=FACE_OUTER_BOUND('',#8879,.T.);
#7240=FACE_OUTER_BOUND('',#8880,.T.);
#7241=FACE_OUTER_BOUND('',#8881,.T.);
#7242=FACE_OUTER_BOUND('',#8882,.T.);
#7243=FACE_OUTER_BOUND('',#8883,.T.);
#7244=FACE_OUTER_BOUND('',#8884,.T.);
#7245=FACE_OUTER_BOUND('',#8885,.T.);
#7246=FACE_OUTER_BOUND('',#8886,.T.);
#7247=FACE_OUTER_BOUND('',#8887,.T.);
#7248=FACE_OUTER_BOUND('',#8888,.T.);
#7249=FACE_OUTER_BOUND('',#8889,.T.);
#7250=FACE_OUTER_BOUND('',#8890,.T.);
#7251=FACE_OUTER_BOUND('',#8891,.T.);
#7252=FACE_OUTER_BOUND('',#8892,.T.);
#7253=FACE_OUTER_BOUND('',#8894,.T.);
#7254=FACE_OUTER_BOUND('',#8895,.T.);
#7255=FACE_OUTER_BOUND('',#8896,.T.);
#7256=FACE_OUTER_BOUND('',#8897,.T.);
#7257=FACE_OUTER_BOUND('',#8898,.T.);
#7258=FACE_OUTER_BOUND('',#8899,.T.);
#7259=FACE_OUTER_BOUND('',#8900,.T.);
#7260=FACE_OUTER_BOUND('',#8901,.T.);
#7261=FACE_OUTER_BOUND('',#8902,.T.);
#7262=FACE_OUTER_BOUND('',#8903,.T.);
#7263=FACE_OUTER_BOUND('',#8904,.T.);
#7264=FACE_OUTER_BOUND('',#8905,.T.);
#7265=FACE_OUTER_BOUND('',#8906,.T.);
#7266=FACE_OUTER_BOUND('',#8908,.T.);
#7267=FACE_OUTER_BOUND('',#8909,.T.);
#7268=FACE_OUTER_BOUND('',#8910,.T.);
#7269=FACE_OUTER_BOUND('',#8911,.T.);
#7270=FACE_OUTER_BOUND('',#8912,.T.);
#7271=FACE_OUTER_BOUND('',#8913,.T.);
#7272=FACE_OUTER_BOUND('',#8914,.T.);
#7273=FACE_OUTER_BOUND('',#8915,.T.);
#7274=FACE_OUTER_BOUND('',#8916,.T.);
#7275=FACE_OUTER_BOUND('',#8917,.T.);
#7276=FACE_OUTER_BOUND('',#8918,.T.);
#7277=FACE_OUTER_BOUND('',#8919,.T.);
#7278=FACE_OUTER_BOUND('',#8921,.T.);
#7279=FACE_OUTER_BOUND('',#8922,.T.);
#7280=FACE_OUTER_BOUND('',#8923,.T.);
#7281=FACE_OUTER_BOUND('',#8924,.T.);
#7282=FACE_OUTER_BOUND('',#8925,.T.);
#7283=FACE_OUTER_BOUND('',#8926,.T.);
#7284=FACE_OUTER_BOUND('',#8927,.T.);
#7285=FACE_OUTER_BOUND('',#8928,.T.);
#7286=FACE_OUTER_BOUND('',#8929,.T.);
#7287=FACE_OUTER_BOUND('',#8930,.T.);
#7288=FACE_OUTER_BOUND('',#8931,.T.);
#7289=FACE_OUTER_BOUND('',#8932,.T.);
#7290=FACE_OUTER_BOUND('',#8934,.T.);
#7291=FACE_OUTER_BOUND('',#8935,.T.);
#7292=FACE_OUTER_BOUND('',#8936,.T.);
#7293=FACE_OUTER_BOUND('',#8937,.T.);
#7294=FACE_OUTER_BOUND('',#8938,.T.);
#7295=FACE_OUTER_BOUND('',#8939,.T.);
#7296=FACE_OUTER_BOUND('',#8940,.T.);
#7297=FACE_OUTER_BOUND('',#8941,.T.);
#7298=FACE_OUTER_BOUND('',#8942,.T.);
#7299=FACE_OUTER_BOUND('',#8943,.T.);
#7300=FACE_OUTER_BOUND('',#8944,.T.);
#7301=FACE_OUTER_BOUND('',#8945,.T.);
#7302=FACE_OUTER_BOUND('',#8946,.T.);
#7303=FACE_OUTER_BOUND('',#8947,.T.);
#7304=FACE_OUTER_BOUND('',#8948,.T.);
#7305=FACE_OUTER_BOUND('',#8949,.T.);
#7306=FACE_OUTER_BOUND('',#8950,.T.);
#7307=FACE_OUTER_BOUND('',#8951,.T.);
#7308=FACE_OUTER_BOUND('',#8952,.T.);
#7309=FACE_OUTER_BOUND('',#8953,.T.);
#7310=FACE_OUTER_BOUND('',#8954,.T.);
#7311=FACE_OUTER_BOUND('',#8955,.T.);
#7312=FACE_OUTER_BOUND('',#8956,.T.);
#7313=FACE_OUTER_BOUND('',#8957,.T.);
#7314=FACE_OUTER_BOUND('',#8958,.T.);
#7315=FACE_OUTER_BOUND('',#8959,.T.);
#7316=FACE_OUTER_BOUND('',#8960,.T.);
#7317=FACE_OUTER_BOUND('',#8961,.T.);
#7318=FACE_OUTER_BOUND('',#8962,.T.);
#7319=FACE_OUTER_BOUND('',#8963,.T.);
#7320=FACE_OUTER_BOUND('',#8964,.T.);
#7321=FACE_OUTER_BOUND('',#8965,.T.);
#7322=FACE_OUTER_BOUND('',#8966,.T.);
#7323=FACE_OUTER_BOUND('',#8967,.T.);
#7324=FACE_OUTER_BOUND('',#8969,.T.);
#7325=FACE_OUTER_BOUND('',#8970,.T.);
#7326=FACE_OUTER_BOUND('',#8972,.T.);
#7327=FACE_OUTER_BOUND('',#8973,.T.);
#7328=FACE_OUTER_BOUND('',#8974,.T.);
#7329=FACE_OUTER_BOUND('',#8975,.T.);
#7330=FACE_OUTER_BOUND('',#8976,.T.);
#7331=FACE_OUTER_BOUND('',#8977,.T.);
#7332=FACE_OUTER_BOUND('',#8978,.T.);
#7333=FACE_OUTER_BOUND('',#8979,.T.);
#7334=FACE_OUTER_BOUND('',#8980,.T.);
#7335=FACE_OUTER_BOUND('',#8981,.T.);
#7336=FACE_OUTER_BOUND('',#8982,.T.);
#7337=FACE_OUTER_BOUND('',#8983,.T.);
#7338=FACE_OUTER_BOUND('',#8984,.T.);
#7339=FACE_OUTER_BOUND('',#8985,.T.);
#7340=FACE_OUTER_BOUND('',#8986,.T.);
#7341=FACE_OUTER_BOUND('',#8987,.T.);
#7342=FACE_OUTER_BOUND('',#8988,.T.);
#7343=FACE_OUTER_BOUND('',#8989,.T.);
#7344=FACE_OUTER_BOUND('',#8990,.T.);
#7345=FACE_OUTER_BOUND('',#8991,.T.);
#7346=FACE_OUTER_BOUND('',#8992,.T.);
#7347=FACE_OUTER_BOUND('',#8993,.T.);
#7348=FACE_OUTER_BOUND('',#8994,.T.);
#8784=EDGE_LOOP('',(#19556,#19557,#19558,#19559));
#8785=EDGE_LOOP('',(#19560,#19561,#19562,#19563));
#8786=EDGE_LOOP('',(#19564,#19565,#19566,#19567,#19568,#19569,#19570,#19571));
#8787=EDGE_LOOP('',(#19572));
#8788=EDGE_LOOP('',(#19573,#19574,#19575,#19576));
#8789=EDGE_LOOP('',(#19577));
#8790=EDGE_LOOP('',(#19578));
#8791=EDGE_LOOP('',(#19579,#19580,#19581,#19582));
#8792=EDGE_LOOP('',(#19583,#19584,#19585,#19586,#19587,#19588,#19589,#19590,
#19591,#19592,#19593));
#8793=EDGE_LOOP('',(#19594));
#8794=EDGE_LOOP('',(#19595,#19596,#19597,#19598,#19599,#19600,#19601,#19602));
#8795=EDGE_LOOP('',(#19603));
#8796=EDGE_LOOP('',(#19604,#19605,#19606,#19607));
#8797=EDGE_LOOP('',(#19608,#19609,#19610,#19611));
#8798=EDGE_LOOP('',(#19612,#19613,#19614,#19615));
#8799=EDGE_LOOP('',(#19616,#19617,#19618,#19619));
#8800=EDGE_LOOP('',(#19620,#19621,#19622,#19623,#19624));
#8801=EDGE_LOOP('',(#19625,#19626,#19627,#19628,#19629,#19630,#19631,#19632,
#19633,#19634,#19635,#19636,#19637));
#8802=EDGE_LOOP('',(#19638,#19639,#19640,#19641,#19642,#19643,#19644,#19645));
#8803=EDGE_LOOP('',(#19646,#19647,#19648,#19649,#19650,#19651));
#8804=EDGE_LOOP('',(#19652,#19653,#19654,#19655,#19656));
#8805=EDGE_LOOP('',(#19657,#19658,#19659,#19660));
#8806=EDGE_LOOP('',(#19661,#19662,#19663,#19664,#19665,#19666,#19667,#19668));
#8807=EDGE_LOOP('',(#19669,#19670,#19671,#19672,#19673,#19674));
#8808=EDGE_LOOP('',(#19675,#19676,#19677,#19678));
#8809=EDGE_LOOP('',(#19679,#19680,#19681,#19682,#19683));
#8810=EDGE_LOOP('',(#19684,#19685,#19686,#19687,#19688,#19689));
#8811=EDGE_LOOP('',(#19690,#19691,#19692,#19693,#19694));
#8812=EDGE_LOOP('',(#19695,#19696,#19697,#19698));
#8813=EDGE_LOOP('',(#19699,#19700,#19701,#19702,#19703,#19704));
#8814=EDGE_LOOP('',(#19705,#19706,#19707,#19708));
#8815=EDGE_LOOP('',(#19709,#19710,#19711,#19712,#19713,#19714,#19715,#19716));
#8816=EDGE_LOOP('',(#19717));
#8817=EDGE_LOOP('',(#19718));
#8818=EDGE_LOOP('',(#19719,#19720,#19721,#19722,#19723,#19724,#19725,#19726));
#8819=EDGE_LOOP('',(#19727));
#8820=EDGE_LOOP('',(#19728));
#8821=EDGE_LOOP('',(#19729,#19730,#19731,#19732));
#8822=EDGE_LOOP('',(#19733,#19734,#19735,#19736));
#8823=EDGE_LOOP('',(#19737,#19738,#19739,#19740));
#8824=EDGE_LOOP('',(#19741,#19742,#19743,#19744));
#8825=EDGE_LOOP('',(#19745));
#8826=EDGE_LOOP('',(#19746));
#8827=EDGE_LOOP('',(#19747));
#8828=EDGE_LOOP('',(#19748));
#8829=EDGE_LOOP('',(#19749));
#8830=EDGE_LOOP('',(#19750));
#8831=EDGE_LOOP('',(#19751,#19752,#19753,#19754));
#8832=EDGE_LOOP('',(#19755,#19756,#19757,#19758));
#8833=EDGE_LOOP('',(#19759,#19760,#19761,#19762));
#8834=EDGE_LOOP('',(#19763,#19764,#19765,#19766));
#8835=EDGE_LOOP('',(#19767,#19768,#19769,#19770));
#8836=EDGE_LOOP('',(#19771,#19772,#19773,#19774));
#8837=EDGE_LOOP('',(#19775,#19776,#19777,#19778));
#8838=EDGE_LOOP('',(#19779,#19780,#19781,#19782));
#8839=EDGE_LOOP('',(#19783,#19784,#19785,#19786,#19787,#19788,#19789,#19790));
#8840=EDGE_LOOP('',(#19791));
#8841=EDGE_LOOP('',(#19792));
#8842=EDGE_LOOP('',(#19793,#19794,#19795,#19796));
#8843=EDGE_LOOP('',(#19797,#19798,#19799,#19800));
#8844=EDGE_LOOP('',(#19801,#19802,#19803,#19804));
#8845=EDGE_LOOP('',(#19805));
#8846=EDGE_LOOP('',(#19806));
#8847=EDGE_LOOP('',(#19807));
#8848=EDGE_LOOP('',(#19808));
#8849=EDGE_LOOP('',(#19809));
#8850=EDGE_LOOP('',(#19810));
#8851=EDGE_LOOP('',(#19811,#19812,#19813,#19814));
#8852=EDGE_LOOP('',(#19815));
#8853=EDGE_LOOP('',(#19816));
#8854=EDGE_LOOP('',(#19817));
#8855=EDGE_LOOP('',(#19818));
#8856=EDGE_LOOP('',(#19819));
#8857=EDGE_LOOP('',(#19820));
#8858=EDGE_LOOP('',(#19821,#19822,#19823,#19824));
#8859=EDGE_LOOP('',(#19825,#19826,#19827,#19828));
#8860=EDGE_LOOP('',(#19829,#19830,#19831,#19832));
#8861=EDGE_LOOP('',(#19833,#19834,#19835,#19836));
#8862=EDGE_LOOP('',(#19837,#19838,#19839,#19840,#19841,#19842,#19843,#19844,
#19845,#19846,#19847,#19848,#19849,#19850,#19851,#19852,#19853,#19854,#19855,
#19856,#19857,#19858));
#8863=EDGE_LOOP('',(#19859,#19860,#19861,#19862));
#8864=EDGE_LOOP('',(#19863,#19864));
#8865=EDGE_LOOP('',(#19865,#19866,#19867,#19868));
#8866=EDGE_LOOP('',(#19869,#19870));
#8867=EDGE_LOOP('',(#19871,#19872,#19873,#19874));
#8868=EDGE_LOOP('',(#19875,#19876));
#8869=EDGE_LOOP('',(#19877,#19878,#19879,#19880));
#8870=EDGE_LOOP('',(#19881,#19882,#19883,#19884));
#8871=EDGE_LOOP('',(#19885,#19886,#19887,#19888));
#8872=EDGE_LOOP('',(#19889,#19890,#19891,#19892));
#8873=EDGE_LOOP('',(#19893,#19894,#19895,#19896));
#8874=EDGE_LOOP('',(#19897,#19898,#19899,#19900));
#8875=EDGE_LOOP('',(#19901,#19902,#19903,#19904));
#8876=EDGE_LOOP('',(#19905,#19906,#19907,#19908));
#8877=EDGE_LOOP('',(#19909,#19910,#19911,#19912));
#8878=EDGE_LOOP('',(#19913,#19914,#19915,#19916,#19917));
#8879=EDGE_LOOP('',(#19918,#19919,#19920,#19921));
#8880=EDGE_LOOP('',(#19922,#19923,#19924,#19925));
#8881=EDGE_LOOP('',(#19926,#19927,#19928,#19929));
#8882=EDGE_LOOP('',(#19930,#19931,#19932,#19933,#19934,#19935));
#8883=EDGE_LOOP('',(#19936,#19937,#19938,#19939,#19940,#19941,#19942));
#8884=EDGE_LOOP('',(#19943,#19944,#19945,#19946));
#8885=EDGE_LOOP('',(#19947,#19948,#19949,#19950));
#8886=EDGE_LOOP('',(#19951,#19952,#19953,#19954));
#8887=EDGE_LOOP('',(#19955,#19956,#19957,#19958));
#8888=EDGE_LOOP('',(#19959,#19960,#19961,#19962));
#8889=EDGE_LOOP('',(#19963,#19964,#19965,#19966,#19967));
#8890=EDGE_LOOP('',(#19968,#19969,#19970,#19971,#19972));
#8891=EDGE_LOOP('',(#19973,#19974,#19975,#19976));
#8892=EDGE_LOOP('',(#19977));
#8893=EDGE_LOOP('',(#19978));
#8894=EDGE_LOOP('',(#19979,#19980,#19981,#19982));
#8895=EDGE_LOOP('',(#19983,#19984,#19985,#19986));
#8896=EDGE_LOOP('',(#19987,#19988,#19989,#19990));
#8897=EDGE_LOOP('',(#19991,#19992,#19993,#19994));
#8898=EDGE_LOOP('',(#19995,#19996,#19997,#19998));
#8899=EDGE_LOOP('',(#19999,#20000,#20001,#20002));
#8900=EDGE_LOOP('',(#20003,#20004,#20005,#20006));
#8901=EDGE_LOOP('',(#20007,#20008,#20009,#20010));
#8902=EDGE_LOOP('',(#20011,#20012,#20013,#20014));
#8903=EDGE_LOOP('',(#20015,#20016,#20017,#20018));
#8904=EDGE_LOOP('',(#20019,#20020,#20021,#20022));
#8905=EDGE_LOOP('',(#20023,#20024,#20025,#20026));
#8906=EDGE_LOOP('',(#20027,#20028,#20029,#20030,#20031,#20032,#20033,#20034));
#8907=EDGE_LOOP('',(#20035,#20036,#20037,#20038,#20039,#20040,#20041,#20042));
#8908=EDGE_LOOP('',(#20043,#20044,#20045,#20046));
#8909=EDGE_LOOP('',(#20047,#20048,#20049,#20050));
#8910=EDGE_LOOP('',(#20051,#20052,#20053,#20054));
#8911=EDGE_LOOP('',(#20055,#20056,#20057,#20058));
#8912=EDGE_LOOP('',(#20059,#20060,#20061,#20062));
#8913=EDGE_LOOP('',(#20063,#20064,#20065,#20066));
#8914=EDGE_LOOP('',(#20067,#20068,#20069,#20070));
#8915=EDGE_LOOP('',(#20071,#20072,#20073,#20074));
#8916=EDGE_LOOP('',(#20075,#20076,#20077,#20078));
#8917=EDGE_LOOP('',(#20079,#20080,#20081,#20082));
#8918=EDGE_LOOP('',(#20083,#20084,#20085,#20086));
#8919=EDGE_LOOP('',(#20087,#20088,#20089,#20090,#20091));
#8920=EDGE_LOOP('',(#20092,#20093,#20094,#20095,#20096,#20097,#20098,#20099));
#8921=EDGE_LOOP('',(#20100,#20101,#20102,#20103));
#8922=EDGE_LOOP('',(#20104,#20105,#20106,#20107));
#8923=EDGE_LOOP('',(#20108,#20109,#20110,#20111));
#8924=EDGE_LOOP('',(#20112,#20113,#20114,#20115));
#8925=EDGE_LOOP('',(#20116,#20117,#20118,#20119));
#8926=EDGE_LOOP('',(#20120,#20121,#20122,#20123));
#8927=EDGE_LOOP('',(#20124,#20125,#20126,#20127));
#8928=EDGE_LOOP('',(#20128,#20129,#20130,#20131));
#8929=EDGE_LOOP('',(#20132,#20133,#20134,#20135));
#8930=EDGE_LOOP('',(#20136,#20137,#20138,#20139,#20140,#20141,#20142,#20143,
#20144,#20145,#20146,#20147));
#8931=EDGE_LOOP('',(#20148,#20149,#20150,#20151));
#8932=EDGE_LOOP('',(#20152,#20153,#20154,#20155,#20156,#20157,#20158,#20159));
#8933=EDGE_LOOP('',(#20160));
#8934=EDGE_LOOP('',(#20161,#20162,#20163,#20164));
#8935=EDGE_LOOP('',(#20165,#20166,#20167,#20168));
#8936=EDGE_LOOP('',(#20169,#20170,#20171,#20172));
#8937=EDGE_LOOP('',(#20173,#20174,#20175,#20176));
#8938=EDGE_LOOP('',(#20177,#20178,#20179,#20180));
#8939=EDGE_LOOP('',(#20181,#20182,#20183,#20184));
#8940=EDGE_LOOP('',(#20185,#20186,#20187,#20188));
#8941=EDGE_LOOP('',(#20189,#20190,#20191,#20192));
#8942=EDGE_LOOP('',(#20193,#20194,#20195,#20196));
#8943=EDGE_LOOP('',(#20197,#20198,#20199,#20200));
#8944=EDGE_LOOP('',(#20201,#20202,#20203,#20204));
#8945=EDGE_LOOP('',(#20205,#20206,#20207,#20208));
#8946=EDGE_LOOP('',(#20209,#20210,#20211,#20212));
#8947=EDGE_LOOP('',(#20213,#20214,#20215,#20216));
#8948=EDGE_LOOP('',(#20217,#20218,#20219,#20220));
#8949=EDGE_LOOP('',(#20221,#20222,#20223,#20224));
#8950=EDGE_LOOP('',(#20225,#20226,#20227,#20228));
#8951=EDGE_LOOP('',(#20229,#20230,#20231,#20232));
#8952=EDGE_LOOP('',(#20233,#20234,#20235,#20236));
#8953=EDGE_LOOP('',(#20237,#20238,#20239,#20240));
#8954=EDGE_LOOP('',(#20241,#20242,#20243,#20244));
#8955=EDGE_LOOP('',(#20245,#20246,#20247,#20248));
#8956=EDGE_LOOP('',(#20249,#20250,#20251,#20252));
#8957=EDGE_LOOP('',(#20253));
#8958=EDGE_LOOP('',(#20254));
#8959=EDGE_LOOP('',(#20255));
#8960=EDGE_LOOP('',(#20256));
#8961=EDGE_LOOP('',(#20257,#20258,#20259,#20260));
#8962=EDGE_LOOP('',(#20261,#20262,#20263,#20264));
#8963=EDGE_LOOP('',(#20265,#20266,#20267,#20268));
#8964=EDGE_LOOP('',(#20269,#20270,#20271,#20272));
#8965=EDGE_LOOP('',(#20273,#20274,#20275,#20276));
#8966=EDGE_LOOP('',(#20277,#20278,#20279,#20280));
#8967=EDGE_LOOP('',(#20281));
#8968=EDGE_LOOP('',(#20282));
#8969=EDGE_LOOP('',(#20283,#20284,#20285,#20286));
#8970=EDGE_LOOP('',(#20287));
#8971=EDGE_LOOP('',(#20288));
#8972=EDGE_LOOP('',(#20289,#20290,#20291,#20292));
#8973=EDGE_LOOP('',(#20293,#20294,#20295,#20296));
#8974=EDGE_LOOP('',(#20297,#20298,#20299,#20300,#20301));
#8975=EDGE_LOOP('',(#20302,#20303,#20304,#20305,#20306,#20307,#20308,#20309));
#8976=EDGE_LOOP('',(#20310,#20311,#20312,#20313,#20314));
#8977=EDGE_LOOP('',(#20315,#20316,#20317,#20318));
#8978=EDGE_LOOP('',(#20319,#20320,#20321,#20322));
#8979=EDGE_LOOP('',(#20323,#20324,#20325,#20326));
#8980=EDGE_LOOP('',(#20327,#20328,#20329,#20330));
#8981=EDGE_LOOP('',(#20331,#20332,#20333,#20334));
#8982=EDGE_LOOP('',(#20335,#20336,#20337,#20338));
#8983=EDGE_LOOP('',(#20339,#20340,#20341,#20342));
#8984=EDGE_LOOP('',(#20343,#20344,#20345,#20346));
#8985=EDGE_LOOP('',(#20347,#20348,#20349,#20350,#20351));
#8986=EDGE_LOOP('',(#20352,#20353,#20354,#20355,#20356));
#8987=EDGE_LOOP('',(#20357,#20358,#20359,#20360,#20361));
#8988=EDGE_LOOP('',(#20362,#20363,#20364,#20365));
#8989=EDGE_LOOP('',(#20366,#20367,#20368,#20369));
#8990=EDGE_LOOP('',(#20370,#20371,#20372,#20373,#20374,#20375,#20376,#20377));
#8991=EDGE_LOOP('',(#20378,#20379,#20380,#20381));
#8992=EDGE_LOOP('',(#20382,#20383,#20384,#20385));
#8993=EDGE_LOOP('',(#20386,#20387,#20388,#20389));
#8994=EDGE_LOOP('',(#20390,#20391,#20392,#20393));
#10384=CIRCLE('',#27991,26.51);
#10385=CIRCLE('',#27992,26.01);
#10386=CIRCLE('',#27994,26.01);
#10387=CIRCLE('',#27996,6.00000000000002);
#10388=CIRCLE('',#27997,6.00000000000002);
#10389=CIRCLE('',#27998,6.00000000000002);
#10390=CIRCLE('',#27999,6.00000000000002);
#10391=CIRCLE('',#28001,26.51);
#10392=CIRCLE('',#28003,27.5);
#10393=CIRCLE('',#28005,7.5);
#10394=CIRCLE('',#28006,7.);
#10395=CIRCLE('',#28008,4.);
#10396=CIRCLE('',#28009,3.99999999999999);
#10397=CIRCLE('',#28010,4.);
#10398=CIRCLE('',#28011,3.99999999999999);
#10399=CIRCLE('',#28012,7.5);
#10400=CIRCLE('',#28013,3.99999999999998);
#10401=CIRCLE('',#28014,3.99999999999999);
#10402=CIRCLE('',#28015,3.99999999999998);
#10403=CIRCLE('',#28016,3.99999999999999);
#10404=CIRCLE('',#28018,7.);
#10405=CIRCLE('',#28020,7.);
#10406=CIRCLE('',#28022,7.);
#10407=CIRCLE('',#28024,2.55);
#10408=CIRCLE('',#28025,3.05);
#10409=CIRCLE('',#28027,3.05);
#10410=CIRCLE('',#28028,3.05);
#10411=CIRCLE('',#28029,3.05);
#10412=CIRCLE('',#28030,7.99999999999999);
#10413=CIRCLE('',#28031,8.00000000000001);
#10414=CIRCLE('',#28032,8.00000000000001);
#10415=CIRCLE('',#28033,7.99999999999998);
#10416=CIRCLE('',#28035,2.55);
#10417=CIRCLE('',#28037,2.55);
#10418=CIRCLE('',#28038,2.55);
#10419=CIRCLE('',#28040,6.00000000000002);
#10420=CIRCLE('',#28042,2.55);
#10421=CIRCLE('',#28044,2.55);
#10422=CIRCLE('',#28046,2.55);
#10423=CIRCLE('',#28048,2.55);
#10424=CIRCLE('',#28049,2.55);
#10425=CIRCLE('',#28051,2.55);
#10426=CIRCLE('',#28053,3.05);
#10427=CIRCLE('',#28055,3.05);
#10428=CIRCLE('',#28056,3.05);
#10429=CIRCLE('',#28057,7.99999999999998);
#10430=CIRCLE('',#28058,8.00000000000001);
#10431=CIRCLE('',#28059,8.00000000000001);
#10432=CIRCLE('',#28060,7.99999999999999);
#10433=CIRCLE('',#28061,3.05);
#10434=CIRCLE('',#28066,7.5);
#10435=CIRCLE('',#28067,7.);
#10436=CIRCLE('',#28069,123.);
#10437=CIRCLE('',#28070,7.5);
#10438=CIRCLE('',#28071,7.5);
#10439=CIRCLE('',#28072,92.1);
#10440=CIRCLE('',#28073,7.50000000000001);
#10441=CIRCLE('',#28075,7.);
#10442=CIRCLE('',#28077,7.);
#10443=CIRCLE('',#28079,7.);
#10444=CIRCLE('',#28081,7.);
#10445=CIRCLE('',#28083,7.);
#10446=CIRCLE('',#28085,6.99999999999999);
#10447=CIRCLE('',#28087,6.99999999999999);
#10448=CIRCLE('',#28089,7.5);
#10449=CIRCLE('',#28091,1.99999999999999);
#10450=CIRCLE('',#28092,2.);
#10451=CIRCLE('',#28093,1.99999999999999);
#10452=CIRCLE('',#28094,2.);
#10453=CIRCLE('',#28095,7.5);
#10454=CIRCLE('',#28098,70.);
#10455=CIRCLE('',#28099,2.);
#10456=CIRCLE('',#28100,68.);
#10457=CIRCLE('',#28102,70.);
#10458=CIRCLE('',#28104,5.5);
#10459=CIRCLE('',#28105,5.5);
#10460=CIRCLE('',#28106,5.5);
#10461=CIRCLE('',#28107,5.5);
#10462=CIRCLE('',#28108,45.);
#10463=CIRCLE('',#28110,2.);
#10464=CIRCLE('',#28111,68.);
#10465=CIRCLE('',#28113,22.5);
#10466=CIRCLE('',#28114,5.5);
#10467=CIRCLE('',#28115,5.5);
#10468=CIRCLE('',#28116,5.5);
#10469=CIRCLE('',#28117,5.5);
#10470=CIRCLE('',#28119,124.428189413237);
#10471=CIRCLE('',#28120,2.);
#10472=CIRCLE('',#28121,123.40620812114);
#10473=CIRCLE('',#28123,119.131441995709);
#10474=CIRCLE('',#28125,125.);
#10475=CIRCLE('',#28127,2.);
#10476=CIRCLE('',#28128,118.866225531784);
#10477=CIRCLE('',#28130,79.7142857142859);
#10478=CIRCLE('',#28131,64.06344373784);
#10479=CIRCLE('',#28132,64.06344373784);
#10480=CIRCLE('',#28133,64.06344373784);
#10481=CIRCLE('',#28134,79.7142857142859);
#10482=CIRCLE('',#28136,63.9364279314891);
#10483=CIRCLE('',#28139,63.9364279314891);
#10484=CIRCLE('',#28142,63.9364279314891);
#10485=CIRCLE('',#28145,1.99999999999998);
#10486=CIRCLE('',#28146,1.99999999999999);
#10487=CIRCLE('',#28147,1.99999999999999);
#10488=CIRCLE('',#28148,4.);
#10489=CIRCLE('',#28150,1.99999999999999);
#10490=CIRCLE('',#28151,1.99999999999999);
#10491=CIRCLE('',#28152,3.99999999999999);
#10492=CIRCLE('',#28154,1.99999999999999);
#10493=CIRCLE('',#28155,1.99999999999999);
#10494=CIRCLE('',#28156,4.);
#10495=CIRCLE('',#28158,1.99999999999999);
#10496=CIRCLE('',#28159,3.99999999999999);
#10497=CIRCLE('',#28165,2.);
#10498=CIRCLE('',#28166,125.);
#10499=CIRCLE('',#28169,47.);
#10500=CIRCLE('',#28170,2.);
#10501=CIRCLE('',#28171,45.);
#10502=CIRCLE('',#28172,47.);
#10503=CIRCLE('',#28173,47.);
#10504=CIRCLE('',#28174,47.);
#10505=CIRCLE('',#28176,6.00000000000002);
#10506=CIRCLE('',#28178,6.00000000000002);
#10507=CIRCLE('',#28181,6.00000000000002);
#10508=CIRCLE('',#28183,45.);
#10509=CIRCLE('',#28185,2.);
#10510=CIRCLE('',#28186,90.1);
#10511=CIRCLE('',#28187,90.1);
#10512=CIRCLE('',#28189,90.1);
#10513=CIRCLE('',#28191,2.);
#10514=CIRCLE('',#28192,47.);
#10515=CIRCLE('',#28195,1.99999999999999);
#10516=CIRCLE('',#28196,2.00000000000001);
#10517=CIRCLE('',#28198,1.99999999999999);
#10518=CIRCLE('',#28199,7.99999999999998);
#10519=CIRCLE('',#28200,5.99999999999998);
#10520=CIRCLE('',#28202,1.99999999999999);
#10521=CIRCLE('',#28204,2.);
#10522=CIRCLE('',#28205,7.99999999999999);
#10523=CIRCLE('',#28206,5.99999999999999);
#10524=CIRCLE('',#28208,2.);
#10525=CIRCLE('',#28210,1.99999999999999);
#10526=CIRCLE('',#28211,8.00000000000001);
#10527=CIRCLE('',#28212,6.00000000000001);
#10528=CIRCLE('',#28214,1.99999999999999);
#10529=CIRCLE('',#28216,8.00000000000001);
#10530=CIRCLE('',#28217,6.00000000000001);
#10531=CIRCLE('',#28219,5.99999999999999);
#10532=CIRCLE('',#28222,5.99999999999998);
#10533=CIRCLE('',#28226,2.);
#10534=CIRCLE('',#28227,2.);
#10535=CIRCLE('',#28229,1.99999999999999);
#10536=CIRCLE('',#28230,8.00000000000001);
#10537=CIRCLE('',#28231,6.00000000000001);
#10538=CIRCLE('',#28233,1.99999999999999);
#10539=CIRCLE('',#28235,2.);
#10540=CIRCLE('',#28236,8.00000000000001);
#10541=CIRCLE('',#28237,6.00000000000001);
#10542=CIRCLE('',#28239,2.);
#10543=CIRCLE('',#28241,1.99999999999999);
#10544=CIRCLE('',#28242,7.99999999999999);
#10545=CIRCLE('',#28244,1.99999999999999);
#10546=CIRCLE('',#28246,7.99999999999998);
#10547=CIRCLE('',#28252,1.99999999999999);
#10548=CIRCLE('',#28253,2.);
#10549=CIRCLE('',#28255,2.);
#10550=CIRCLE('',#28256,6.);
#10551=CIRCLE('',#28257,8.);
#10552=CIRCLE('',#28259,2.);
#10553=CIRCLE('',#28261,2.);
#10554=CIRCLE('',#28262,6.);
#10555=CIRCLE('',#28263,8.);
#10556=CIRCLE('',#28265,2.);
#10557=CIRCLE('',#28267,2.);
#10558=CIRCLE('',#28268,6.);
#10559=CIRCLE('',#28269,8.);
#10560=CIRCLE('',#28271,2.);
#10561=CIRCLE('',#28273,8.);
#10562=CIRCLE('',#28274,6.);
#10563=CIRCLE('',#28277,3.99999999999999);
#10564=CIRCLE('',#28278,3.99999999999998);
#10565=CIRCLE('',#28279,3.99999999999999);
#10566=CIRCLE('',#28280,3.99999999999998);
#10567=CIRCLE('',#28283,40.2777777777778);
#10568=CIRCLE('',#28285,1.99999999999999);
#10569=CIRCLE('',#28286,1.99999999999999);
#10570=CIRCLE('',#28288,2.);
#10571=CIRCLE('',#28289,5.99999999999998);
#10572=CIRCLE('',#28291,2.);
#10573=CIRCLE('',#28293,1.99999999999999);
#10574=CIRCLE('',#28294,6.00000000000001);
#10575=CIRCLE('',#28296,1.99999999999999);
#10576=CIRCLE('',#28298,2.);
#10577=CIRCLE('',#28299,6.00000000000001);
#10578=CIRCLE('',#28301,2.);
#10579=CIRCLE('',#28303,5.99999999999999);
#10580=CIRCLE('',#28305,6.00000000000001);
#10581=CIRCLE('',#28308,5.99999999999998);
#10582=CIRCLE('',#28311,2.);
#10583=CIRCLE('',#28312,1.99999999999999);
#10584=CIRCLE('',#28314,2.);
#10585=CIRCLE('',#28315,5.99999999999999);
#10586=CIRCLE('',#28317,2.);
#10587=CIRCLE('',#28319,1.99999999999999);
#10588=CIRCLE('',#28320,6.00000000000001);
#10589=CIRCLE('',#28322,1.99999999999999);
#10590=CIRCLE('',#28324,2.);
#10591=CIRCLE('',#28326,2.00000000000001);
#10592=CIRCLE('',#28342,27.5);
#10593=CIRCLE('',#28343,26.01);
#10594=CIRCLE('',#28346,26.01);
#10595=CIRCLE('',#28347,22.5);
#11167=B_SPLINE_CURVE_WITH_KNOTS('',3,(#41609,#41610,#41611,#41612),
 .UNSPECIFIED.,.F.,.F.,(4,4),(2.9602728791883,3.32291242799128),
 .UNSPECIFIED.);
#11168=B_SPLINE_CURVE_WITH_KNOTS('',3,(#41614,#41615,#41616,#41617),
 .UNSPECIFIED.,.F.,.F.,(4,4),(-3.32291242799128,-3.14159265358979),
 .UNSPECIFIED.);
#11169=B_SPLINE_CURVE_WITH_KNOTS('',3,(#41618,#41619,#41620,#41621),
 .UNSPECIFIED.,.F.,.F.,(4,4),(-3.14159265358979,-2.9602728791883),
 .UNSPECIFIED.);
#11170=B_SPLINE_CURVE_WITH_KNOTS('',3,(#41687,#41688,#41689,#41690),
 .UNSPECIFIED.,.F.,.F.,(4,4),(-0.181319774401493,0.181319774401488),
 .UNSPECIFIED.);
#11171=B_SPLINE_CURVE_WITH_KNOTS('',3,(#41691,#41692,#41693,#41694),
 .UNSPECIFIED.,.F.,.F.,(4,4),(-0.181319774401488,0.181319774401493),
 .UNSPECIFIED.);
#11172=B_SPLINE_CURVE_WITH_KNOTS('',3,(#41699,#41700,#41701,#41702),
 .UNSPECIFIED.,.F.,.F.,(4,4),(6.10186553277809,6.46450508158109),
 .UNSPECIFIED.);
#11173=B_SPLINE_CURVE_WITH_KNOTS('',3,(#41729,#41730,#41731,#41732),
 .UNSPECIFIED.,.F.,.F.,(4,4),(2.9602728791883,3.32291242799128),
 .UNSPECIFIED.);
#11174=B_SPLINE_CURVE_WITH_KNOTS('',3,(#41734,#41735,#41736,#41737),
 .UNSPECIFIED.,.F.,.F.,(4,4),(-3.32291242799128,-3.14159265358979),
 .UNSPECIFIED.);
#11175=B_SPLINE_CURVE_WITH_KNOTS('',3,(#41738,#41739,#41740,#41741),
 .UNSPECIFIED.,.F.,.F.,(4,4),(-3.14159265358979,-2.9602728791883),
 .UNSPECIFIED.);
#11176=B_SPLINE_CURVE_WITH_KNOTS('',3,(#41770,#41771,#41772,#41773),
 .UNSPECIFIED.,.F.,.F.,(4,4),(-6.46450508158109,-6.10186553277809),
 .UNSPECIFIED.);
#11177=B_SPLINE_CURVE_WITH_KNOTS('',3,(#41793,#41794,#41795,#41796),
 .UNSPECIFIED.,.F.,.F.,(4,4),(0.413605043247719,0.437854341815321),
 .UNSPECIFIED.);
#11178=B_SPLINE_CURVE_WITH_KNOTS('',3,(#41800,#41801,#41802,#41803),
 .UNSPECIFIED.,.F.,.F.,(4,4),(1.36755809423905,1.39180739280665),
 .UNSPECIFIED.);
#11179=B_SPLINE_CURVE_WITH_KNOTS('',3,(#41966,#41967,#41968,#41969,#41970,
#41971,#41972,#41973,#41974,#41975,#41976,#41977,#41978,#41979,#41980,#41981,
#41982,#41983),.UNSPECIFIED.,.F.,.F.,(4,2,2,2,2,2,2,2,4),(2.77896888287132,
2.78150698603454,2.79283731888666,2.85278626064221,2.96447510619432,3.07616395174642,
3.29954164285062,3.83796248419292,4.32657905104996),.UNSPECIFIED.);
#11180=B_SPLINE_CURVE_WITH_KNOTS('',3,(#41988,#41989,#41990,#41991,#41992,
#41993,#41994,#41995,#41996,#41997),.UNSPECIFIED.,.F.,.F.,(4,2,2,2,4),(0.700334773405899,
0.978276696075167,1.30411559546238,1.6299544948496,1.90789641751887),
 .UNSPECIFIED.);
#11181=B_SPLINE_CURVE_WITH_KNOTS('',3,(#42000,#42001,#42002,#42003,#42004,
#42005,#42006,#42007,#42008,#42009),.UNSPECIFIED.,.F.,.F.,(4,2,2,2,4),(0.7003347734059,
0.978276696075167,1.30411559546238,1.6299544948496,1.90789641751887),
 .UNSPECIFIED.);
#11182=B_SPLINE_CURVE_WITH_KNOTS('',3,(#42021,#42022,#42023,#42024,#42025,
#42026,#42027,#42028,#42029,#42030),.UNSPECIFIED.,.F.,.F.,(4,2,2,2,4),(0.700334773405899,
0.978276696075167,1.30411559546238,1.6299544948496,1.90789641751887),
 .UNSPECIFIED.);
#11183=B_SPLINE_CURVE_WITH_KNOTS('',3,(#42042,#42043,#42044,#42045,#42046,
#42047,#42048,#42049,#42050,#42051),.UNSPECIFIED.,.F.,.F.,(4,2,2,2,4),(0.7003347734059,
0.978276696075167,1.30411559546238,1.6299544948496,1.90789641751886),
 .UNSPECIFIED.);
#11184=B_SPLINE_CURVE_WITH_KNOTS('',3,(#42057,#42058,#42059,#42060,#42061,
#42062,#42063,#42064,#42065,#42066,#42067,#42068,#42069,#42070,#42071,#42072,
#42073,#42074),.UNSPECIFIED.,.F.,.F.,(4,2,2,2,2,2,2,2,4),(1.12664595716984,
1.61526252402689,2.15368336536918,2.37706105647338,2.48874990202548,2.60043874757758,
2.66038768933314,2.67171802218525,2.67425612534847),.UNSPECIFIED.);
#11185=B_SPLINE_CURVE_WITH_KNOTS('',3,(#42078,#42079,#42080,#42081),
 .UNSPECIFIED.,.F.,.F.,(4,4),(1.36755809423905,1.39180739280665),
 .UNSPECIFIED.);
#11186=B_SPLINE_CURVE_WITH_KNOTS('',3,(#42084,#42085,#42086,#42087),
 .UNSPECIFIED.,.F.,.F.,(4,4),(0.413605043247719,0.437854341815321),
 .UNSPECIFIED.);
#11187=B_SPLINE_CURVE_WITH_KNOTS('',3,(#42092,#42093,#42094,#42095),
 .UNSPECIFIED.,.F.,.F.,(4,4),(1.36755809423905,1.39180739280665),
 .UNSPECIFIED.);
#11188=B_SPLINE_CURVE_WITH_KNOTS('',3,(#42098,#42099,#42100,#42101),
 .UNSPECIFIED.,.F.,.F.,(4,4),(0.41360504324772,0.437854341815321),
 .UNSPECIFIED.);
#12018=VERTEX_POINT('',#41494);
#12019=VERTEX_POINT('',#41496);
#12020=VERTEX_POINT('',#41500);
#12021=VERTEX_POINT('',#41504);
#12022=VERTEX_POINT('',#41505);
#12023=VERTEX_POINT('',#41507);
#12024=VERTEX_POINT('',#41509);
#12025=VERTEX_POINT('',#41511);
#12026=VERTEX_POINT('',#41513);
#12027=VERTEX_POINT('',#41515);
#12028=VERTEX_POINT('',#41517);
#12029=VERTEX_POINT('',#41521);
#12030=VERTEX_POINT('',#41525);
#12031=VERTEX_POINT('',#41528);
#12032=VERTEX_POINT('',#41530);
#12033=VERTEX_POINT('',#41534);
#12034=VERTEX_POINT('',#41535);
#12035=VERTEX_POINT('',#41537);
#12036=VERTEX_POINT('',#41539);
#12037=VERTEX_POINT('',#41541);
#12038=VERTEX_POINT('',#41543);
#12039=VERTEX_POINT('',#41545);
#12040=VERTEX_POINT('',#41547);
#12041=VERTEX_POINT('',#41549);
#12042=VERTEX_POINT('',#41551);
#12043=VERTEX_POINT('',#41554);
#12044=VERTEX_POINT('',#41556);
#12045=VERTEX_POINT('',#41557);
#12046=VERTEX_POINT('',#41559);
#12047=VERTEX_POINT('',#41561);
#12048=VERTEX_POINT('',#41563);
#12049=VERTEX_POINT('',#41565);
#12050=VERTEX_POINT('',#41567);
#12051=VERTEX_POINT('',#41569);
#12052=VERTEX_POINT('',#41573);
#12053=VERTEX_POINT('',#41577);
#12054=VERTEX_POINT('',#41581);
#12055=VERTEX_POINT('',#41585);
#12056=VERTEX_POINT('',#41586);
#12057=VERTEX_POINT('',#41588);
#12058=VERTEX_POINT('',#41590);
#12059=VERTEX_POINT('',#41613);
#12060=VERTEX_POINT('',#41623);
#12061=VERTEX_POINT('',#41625);
#12062=VERTEX_POINT('',#41628);
#12063=VERTEX_POINT('',#41630);
#12064=VERTEX_POINT('',#41632);
#12065=VERTEX_POINT('',#41634);
#12066=VERTEX_POINT('',#41636);
#12067=VERTEX_POINT('',#41638);
#12068=VERTEX_POINT('',#41640);
#12069=VERTEX_POINT('',#41643);
#12070=VERTEX_POINT('',#41644);
#12071=VERTEX_POINT('',#41646);
#12072=VERTEX_POINT('',#41648);
#12073=VERTEX_POINT('',#41650);
#12074=VERTEX_POINT('',#41652);
#12075=VERTEX_POINT('',#41654);
#12076=VERTEX_POINT('',#41656);
#12077=VERTEX_POINT('',#41660);
#12078=VERTEX_POINT('',#41664);
#12079=VERTEX_POINT('',#41666);
#12080=VERTEX_POINT('',#41668);
#12081=VERTEX_POINT('',#41696);
#12082=VERTEX_POINT('',#41704);
#12083=VERTEX_POINT('',#41708);
#12084=VERTEX_POINT('',#41710);
#12085=VERTEX_POINT('',#41733);
#12086=VERTEX_POINT('',#41743);
#12087=VERTEX_POINT('',#41747);
#12088=VERTEX_POINT('',#41749);
#12089=VERTEX_POINT('',#41751);
#12090=VERTEX_POINT('',#41775);
#12091=VERTEX_POINT('',#41779);
#12092=VERTEX_POINT('',#41783);
#12093=VERTEX_POINT('',#41784);
#12094=VERTEX_POINT('',#41786);
#12095=VERTEX_POINT('',#41788);
#12096=VERTEX_POINT('',#41792);
#12097=VERTEX_POINT('',#41797);
#12098=VERTEX_POINT('',#41799);
#12099=VERTEX_POINT('',#41804);
#12100=VERTEX_POINT('',#41809);
#12101=VERTEX_POINT('',#41811);
#12102=VERTEX_POINT('',#41813);
#12103=VERTEX_POINT('',#41814);
#12104=VERTEX_POINT('',#41816);
#12105=VERTEX_POINT('',#41818);
#12106=VERTEX_POINT('',#41820);
#12107=VERTEX_POINT('',#41822);
#12108=VERTEX_POINT('',#41824);
#12109=VERTEX_POINT('',#41826);
#12110=VERTEX_POINT('',#41829);
#12111=VERTEX_POINT('',#41838);
#12112=VERTEX_POINT('',#41840);
#12113=VERTEX_POINT('',#41844);
#12114=VERTEX_POINT('',#41846);
#12115=VERTEX_POINT('',#41848);
#12116=VERTEX_POINT('',#41850);
#12117=VERTEX_POINT('',#41852);
#12118=VERTEX_POINT('',#41855);
#12119=VERTEX_POINT('',#41859);
#12120=VERTEX_POINT('',#41863);
#12121=VERTEX_POINT('',#41867);
#12122=VERTEX_POINT('',#41871);
#12123=VERTEX_POINT('',#41875);
#12124=VERTEX_POINT('',#41879);
#12125=VERTEX_POINT('',#41883);
#12126=VERTEX_POINT('',#41887);
#12127=VERTEX_POINT('',#41888);
#12128=VERTEX_POINT('',#41890);
#12129=VERTEX_POINT('',#41892);
#12130=VERTEX_POINT('',#41894);
#12131=VERTEX_POINT('',#41896);
#12132=VERTEX_POINT('',#41898);
#12133=VERTEX_POINT('',#41900);
#12134=VERTEX_POINT('',#41903);
#12135=VERTEX_POINT('',#41908);
#12136=VERTEX_POINT('',#41910);
#12137=VERTEX_POINT('',#41914);
#12138=VERTEX_POINT('',#41918);
#12139=VERTEX_POINT('',#41920);
#12140=VERTEX_POINT('',#41922);
#12141=VERTEX_POINT('',#41924);
#12142=VERTEX_POINT('',#41926);
#12143=VERTEX_POINT('',#41929);
#12144=VERTEX_POINT('',#41933);
#12145=VERTEX_POINT('',#41935);
#12146=VERTEX_POINT('',#41937);
#12147=VERTEX_POINT('',#41939);
#12148=VERTEX_POINT('',#41941);
#12149=VERTEX_POINT('',#41944);
#12150=VERTEX_POINT('',#41946);
#12151=VERTEX_POINT('',#41950);
#12152=VERTEX_POINT('',#41957);
#12153=VERTEX_POINT('',#41961);
#12154=VERTEX_POINT('',#41963);
#12155=VERTEX_POINT('',#41965);
#12156=VERTEX_POINT('',#41984);
#12157=VERTEX_POINT('',#41999);
#12158=VERTEX_POINT('',#42010);
#12159=VERTEX_POINT('',#42014);
#12160=VERTEX_POINT('',#42016);
#12161=VERTEX_POINT('',#42020);
#12162=VERTEX_POINT('',#42031);
#12163=VERTEX_POINT('',#42035);
#12164=VERTEX_POINT('',#42037);
#12165=VERTEX_POINT('',#42041);
#12166=VERTEX_POINT('',#42052);
#12167=VERTEX_POINT('',#42056);
#12168=VERTEX_POINT('',#42077);
#12169=VERTEX_POINT('',#42082);
#12170=VERTEX_POINT('',#42091);
#12171=VERTEX_POINT('',#42096);
#12172=VERTEX_POINT('',#42108);
#12173=VERTEX_POINT('',#42110);
#12174=VERTEX_POINT('',#42122);
#12175=VERTEX_POINT('',#42126);
#12176=VERTEX_POINT('',#42138);
#12177=VERTEX_POINT('',#42142);
#12178=VERTEX_POINT('',#42154);
#12179=VERTEX_POINT('',#42158);
#12180=VERTEX_POINT('',#42181);
#12181=VERTEX_POINT('',#42188);
#12182=VERTEX_POINT('',#42190);
#12183=VERTEX_POINT('',#42193);
#12184=VERTEX_POINT('',#42195);
#12185=VERTEX_POINT('',#42199);
#12186=VERTEX_POINT('',#42201);
#12187=VERTEX_POINT('',#42205);
#12188=VERTEX_POINT('',#42207);
#12189=VERTEX_POINT('',#42213);
#12190=VERTEX_POINT('',#42217);
#12191=VERTEX_POINT('',#42221);
#12192=VERTEX_POINT('',#42223);
#12193=VERTEX_POINT('',#42227);
#12194=VERTEX_POINT('',#42231);
#12195=VERTEX_POINT('',#42236);
#12196=VERTEX_POINT('',#42237);
#12197=VERTEX_POINT('',#42239);
#12198=VERTEX_POINT('',#42241);
#12199=VERTEX_POINT('',#42245);
#12200=VERTEX_POINT('',#42246);
#12201=VERTEX_POINT('',#42251);
#12202=VERTEX_POINT('',#42252);
#12203=VERTEX_POINT('',#42257);
#12204=VERTEX_POINT('',#42258);
#12205=VERTEX_POINT('',#42263);
#12206=VERTEX_POINT('',#42264);
#12207=VERTEX_POINT('',#42269);
#12208=VERTEX_POINT('',#42270);
#12209=VERTEX_POINT('',#42275);
#12210=VERTEX_POINT('',#42276);
#12211=VERTEX_POINT('',#42284);
#12212=VERTEX_POINT('',#42286);
#12213=VERTEX_POINT('',#42290);
#12214=VERTEX_POINT('',#42294);
#12215=VERTEX_POINT('',#42298);
#12216=VERTEX_POINT('',#42302);
#12217=VERTEX_POINT('',#42303);
#12218=VERTEX_POINT('',#42308);
#12219=VERTEX_POINT('',#42310);
#12220=VERTEX_POINT('',#42314);
#12221=VERTEX_POINT('',#42315);
#12222=VERTEX_POINT('',#42320);
#12223=VERTEX_POINT('',#42321);
#12224=VERTEX_POINT('',#42326);
#12225=VERTEX_POINT('',#42327);
#12226=VERTEX_POINT('',#42332);
#12227=VERTEX_POINT('',#42337);
#12228=VERTEX_POINT('',#42341);
#12229=VERTEX_POINT('',#42356);
#12230=VERTEX_POINT('',#42358);
#12231=VERTEX_POINT('',#42362);
#12232=VERTEX_POINT('',#42363);
#12233=VERTEX_POINT('',#42368);
#12234=VERTEX_POINT('',#42369);
#12235=VERTEX_POINT('',#42374);
#12236=VERTEX_POINT('',#42379);
#12237=VERTEX_POINT('',#42383);
#12238=VERTEX_POINT('',#42384);
#12239=VERTEX_POINT('',#42389);
#12240=VERTEX_POINT('',#42390);
#12241=VERTEX_POINT('',#42401);
#12242=VERTEX_POINT('',#42403);
#12243=VERTEX_POINT('',#42405);
#12244=VERTEX_POINT('',#42407);
#12245=VERTEX_POINT('',#42409);
#12246=VERTEX_POINT('',#42411);
#12247=VERTEX_POINT('',#42416);
#12248=VERTEX_POINT('',#42419);
#12249=VERTEX_POINT('',#42421);
#12250=VERTEX_POINT('',#42425);
#12251=VERTEX_POINT('',#42429);
#12252=VERTEX_POINT('',#42433);
#12253=VERTEX_POINT('',#42437);
#12254=VERTEX_POINT('',#42441);
#12255=VERTEX_POINT('',#42445);
#12256=VERTEX_POINT('',#42451);
#12257=VERTEX_POINT('',#42453);
#12258=VERTEX_POINT('',#42457);
#12259=VERTEX_POINT('',#42461);
#12260=VERTEX_POINT('',#42465);
#12261=VERTEX_POINT('',#42472);
#12262=VERTEX_POINT('',#42476);
#12263=VERTEX_POINT('',#42480);
#12264=VERTEX_POINT('',#42512);
#12265=VERTEX_POINT('',#42514);
#12266=VERTEX_POINT('',#42519);
#12267=VERTEX_POINT('',#42521);
#14782=EDGE_CURVE('',#12018,#12018,#10384,.T.);
#14783=EDGE_CURVE('',#12018,#12019,#2176,.T.);
#14784=EDGE_CURVE('',#12019,#12019,#10385,.T.);
#14785=EDGE_CURVE('',#12020,#12020,#10386,.T.);
#14786=EDGE_CURVE('',#12020,#12019,#2177,.T.);
#14787=EDGE_CURVE('',#12021,#12022,#10387,.T.);
#14788=EDGE_CURVE('',#12023,#12022,#2178,.T.);
#14789=EDGE_CURVE('',#12023,#12024,#10388,.T.);
#14790=EDGE_CURVE('',#12025,#12024,#2179,.T.);
#14791=EDGE_CURVE('',#12025,#12026,#10389,.T.);
#14792=EDGE_CURVE('',#12027,#12026,#2180,.T.);
#14793=EDGE_CURVE('',#12027,#12028,#10390,.T.);
#14794=EDGE_CURVE('',#12021,#12028,#2181,.T.);
#14795=EDGE_CURVE('',#12020,#12029,#2182,.T.);
#14796=EDGE_CURVE('',#12029,#12029,#10391,.T.);
#14797=EDGE_CURVE('',#12030,#12030,#10392,.T.);
#14798=EDGE_CURVE('',#12031,#12031,#10393,.T.);
#14799=EDGE_CURVE('',#12031,#12032,#2183,.T.);
#14800=EDGE_CURVE('',#12032,#12032,#10394,.T.);
#14801=EDGE_CURVE('',#12033,#12034,#10395,.T.);
#14802=EDGE_CURVE('',#12034,#12035,#2184,.T.);
#14803=EDGE_CURVE('',#12035,#12036,#10396,.T.);
#14804=EDGE_CURVE('',#12036,#12037,#2185,.T.);
#14805=EDGE_CURVE('',#12037,#12038,#10397,.T.);
#14806=EDGE_CURVE('',#12038,#12039,#2186,.T.);
#14807=EDGE_CURVE('',#12040,#12039,#2187,.T.);
#14808=EDGE_CURVE('',#12039,#12041,#2188,.T.);
#14809=EDGE_CURVE('',#12041,#12042,#10398,.T.);
#14810=EDGE_CURVE('',#12042,#12033,#2189,.T.);
#14811=EDGE_CURVE('',#12043,#12043,#10399,.T.);
#14812=EDGE_CURVE('',#12044,#12045,#2190,.T.);
#14813=EDGE_CURVE('',#12046,#12044,#10400,.T.);
#14814=EDGE_CURVE('',#12047,#12046,#2191,.T.);
#14815=EDGE_CURVE('',#12048,#12047,#10401,.T.);
#14816=EDGE_CURVE('',#12049,#12048,#2192,.T.);
#14817=EDGE_CURVE('',#12050,#12049,#10402,.T.);
#14818=EDGE_CURVE('',#12051,#12050,#2193,.T.);
#14819=EDGE_CURVE('',#12045,#12051,#10403,.T.);
#14820=EDGE_CURVE('',#12032,#12052,#2194,.T.);
#14821=EDGE_CURVE('',#12052,#12052,#10404,.T.);
#14822=EDGE_CURVE('',#12043,#12053,#2195,.T.);
#14823=EDGE_CURVE('',#12053,#12053,#10405,.T.);
#14824=EDGE_CURVE('',#12053,#12054,#2196,.T.);
#14825=EDGE_CURVE('',#12054,#12054,#10406,.T.);
#14826=EDGE_CURVE('',#12055,#12056,#2197,.T.);
#14827=EDGE_CURVE('',#12056,#12057,#10407,.T.);
#14828=EDGE_CURVE('',#12057,#12058,#2198,.T.);
#14829=EDGE_CURVE('',#12058,#12055,#10408,.T.);
#14830=EDGE_CURVE('',#12055,#12058,#11167,.T.);
#14831=EDGE_CURVE('',#12057,#12059,#11168,.T.);
#14832=EDGE_CURVE('',#12059,#12056,#11169,.T.);
#14833=EDGE_CURVE('',#12060,#12058,#2199,.T.);
#14834=EDGE_CURVE('',#12061,#12060,#10409,.T.);
#14835=EDGE_CURVE('',#12025,#12061,#2200,.T.);
#14836=EDGE_CURVE('',#12024,#12062,#2201,.T.);
#14837=EDGE_CURVE('',#12063,#12062,#10410,.T.);
#14838=EDGE_CURVE('',#12063,#12064,#2202,.T.);
#14839=EDGE_CURVE('',#12065,#12064,#10411,.T.);
#14840=EDGE_CURVE('',#12065,#12066,#2203,.T.);
#14841=EDGE_CURVE('',#12066,#12067,#2204,.T.);
#14842=EDGE_CURVE('',#12067,#12068,#2205,.T.);
#14843=EDGE_CURVE('',#12055,#12068,#2206,.T.);
#14844=EDGE_CURVE('',#12069,#12070,#2207,.T.);
#14845=EDGE_CURVE('',#12071,#12069,#10412,.T.);
#14846=EDGE_CURVE('',#12072,#12071,#2208,.T.);
#14847=EDGE_CURVE('',#12073,#12072,#10413,.T.);
#14848=EDGE_CURVE('',#12074,#12073,#2209,.T.);
#14849=EDGE_CURVE('',#12075,#12074,#10414,.T.);
#14850=EDGE_CURVE('',#12076,#12075,#2210,.T.);
#14851=EDGE_CURVE('',#12070,#12076,#10415,.T.);
#14852=EDGE_CURVE('',#12077,#12077,#10416,.T.);
#14853=EDGE_CURVE('',#12077,#12059,#2211,.T.);
#14854=EDGE_CURVE('',#12062,#12078,#2212,.T.);
#14855=EDGE_CURVE('',#12078,#12079,#10417,.T.);
#14856=EDGE_CURVE('',#12079,#12080,#10418,.T.);
#14857=EDGE_CURVE('',#12080,#12063,#2213,.T.);
#14858=EDGE_CURVE('',#12062,#12063,#11170,.T.);
#14859=EDGE_CURVE('',#12080,#12078,#11171,.T.);
#14860=EDGE_CURVE('',#12023,#12081,#2214,.T.);
#14861=EDGE_CURVE('',#12081,#12066,#10419,.T.);
#14862=EDGE_CURVE('',#12064,#12065,#11172,.T.);
#14863=EDGE_CURVE('',#12082,#12082,#10420,.T.);
#14864=EDGE_CURVE('',#12082,#12079,#2215,.T.);
#14865=EDGE_CURVE('',#12060,#12083,#2216,.T.);
#14866=EDGE_CURVE('',#12083,#12084,#10421,.T.);
#14867=EDGE_CURVE('',#12084,#12061,#2217,.T.);
#14868=EDGE_CURVE('',#12060,#12061,#11173,.T.);
#14869=EDGE_CURVE('',#12084,#12085,#11174,.T.);
#14870=EDGE_CURVE('',#12085,#12083,#11175,.T.);
#14871=EDGE_CURVE('',#12086,#12086,#10422,.T.);
#14872=EDGE_CURVE('',#12086,#12085,#2218,.T.);
#14873=EDGE_CURVE('',#12064,#12087,#2219,.T.);
#14874=EDGE_CURVE('',#12087,#12088,#10423,.T.);
#14875=EDGE_CURVE('',#12088,#12089,#10424,.T.);
#14876=EDGE_CURVE('',#12089,#12065,#2220,.T.);
#14877=EDGE_CURVE('',#12089,#12087,#11176,.T.);
#14878=EDGE_CURVE('',#12090,#12090,#10425,.T.);
#14879=EDGE_CURVE('',#12090,#12088,#2221,.T.);
#14880=EDGE_CURVE('',#12091,#12091,#10426,.T.);
#14881=EDGE_CURVE('',#12091,#12090,#2222,.T.);
#14882=EDGE_CURVE('',#12092,#12093,#2223,.T.);
#14883=EDGE_CURVE('',#12092,#12094,#2224,.T.);
#14884=EDGE_CURVE('',#12094,#12095,#155,.T.);
#14885=EDGE_CURVE('',#12096,#12095,#11177,.F.);
#14886=EDGE_CURVE('',#12096,#12097,#2225,.T.);
#14887=EDGE_CURVE('',#12098,#12097,#11178,.F.);
#14888=EDGE_CURVE('',#12098,#12099,#156,.T.);
#14889=EDGE_CURVE('',#12093,#12099,#2226,.T.);
#14890=EDGE_CURVE('',#12100,#12100,#10427,.T.);
#14891=EDGE_CURVE('',#12101,#12101,#10428,.T.);
#14892=EDGE_CURVE('',#12102,#12103,#2227,.T.);
#14893=EDGE_CURVE('',#12104,#12102,#10429,.T.);
#14894=EDGE_CURVE('',#12105,#12104,#2228,.T.);
#14895=EDGE_CURVE('',#12106,#12105,#10430,.T.);
#14896=EDGE_CURVE('',#12107,#12106,#2229,.T.);
#14897=EDGE_CURVE('',#12108,#12107,#10431,.T.);
#14898=EDGE_CURVE('',#12109,#12108,#2230,.T.);
#14899=EDGE_CURVE('',#12103,#12109,#10432,.T.);
#14900=EDGE_CURVE('',#12110,#12110,#10433,.T.);
#14901=EDGE_CURVE('',#12100,#12086,#2231,.T.);
#14902=EDGE_CURVE('',#12110,#12082,#2232,.T.);
#14903=EDGE_CURVE('',#12101,#12077,#2233,.T.);
#14904=EDGE_CURVE('',#12111,#12111,#10434,.T.);
#14905=EDGE_CURVE('',#12111,#12112,#2234,.T.);
#14906=EDGE_CURVE('',#12112,#12112,#10435,.T.);
#14907=EDGE_CURVE('',#12113,#12113,#10436,.T.);
#14908=EDGE_CURVE('',#12114,#12114,#10437,.T.);
#14909=EDGE_CURVE('',#12115,#12115,#10438,.T.);
#14910=EDGE_CURVE('',#12116,#12116,#10439,.T.);
#14911=EDGE_CURVE('',#12117,#12117,#10440,.T.);
#14912=EDGE_CURVE('',#12118,#12118,#10441,.T.);
#14913=EDGE_CURVE('',#12118,#12112,#2235,.T.);
#14914=EDGE_CURVE('',#12114,#12119,#2236,.T.);
#14915=EDGE_CURVE('',#12119,#12119,#10442,.T.);
#14916=EDGE_CURVE('',#12120,#12120,#10443,.T.);
#14917=EDGE_CURVE('',#12120,#12119,#2237,.T.);
#14918=EDGE_CURVE('',#12117,#12121,#2238,.T.);
#14919=EDGE_CURVE('',#12121,#12121,#10444,.T.);
#14920=EDGE_CURVE('',#12122,#12122,#10445,.T.);
#14921=EDGE_CURVE('',#12122,#12121,#2239,.T.);
#14922=EDGE_CURVE('',#12115,#12123,#2240,.T.);
#14923=EDGE_CURVE('',#12123,#12123,#10446,.T.);
#14924=EDGE_CURVE('',#12124,#12124,#10447,.T.);
#14925=EDGE_CURVE('',#12124,#12123,#2241,.T.);
#14926=EDGE_CURVE('',#12125,#12125,#10448,.T.);
#14927=EDGE_CURVE('',#12125,#12054,#2242,.T.);
#14928=EDGE_CURVE('',#12126,#12127,#2243,.T.);
#14929=EDGE_CURVE('',#12128,#12126,#10449,.T.);
#14930=EDGE_CURVE('',#12129,#12128,#2244,.T.);
#14931=EDGE_CURVE('',#12130,#12129,#10450,.T.);
#14932=EDGE_CURVE('',#12131,#12130,#2245,.T.);
#14933=EDGE_CURVE('',#12132,#12131,#10451,.T.);
#14934=EDGE_CURVE('',#12133,#12132,#2246,.T.);
#14935=EDGE_CURVE('',#12127,#12133,#10452,.T.);
#14936=EDGE_CURVE('',#12134,#12134,#10453,.T.);
#14937=EDGE_CURVE('',#12134,#12052,#2247,.T.);
#14938=EDGE_CURVE('',#12135,#12135,#10454,.T.);
#14939=EDGE_CURVE('',#12135,#12136,#10455,.T.);
#14940=EDGE_CURVE('',#12136,#12136,#10456,.T.);
#14941=EDGE_CURVE('',#12135,#12137,#2248,.T.);
#14942=EDGE_CURVE('',#12137,#12137,#10457,.T.);
#14943=EDGE_CURVE('',#12138,#12138,#10458,.T.);
#14944=EDGE_CURVE('',#12139,#12139,#10459,.T.);
#14945=EDGE_CURVE('',#12140,#12140,#10460,.T.);
#14946=EDGE_CURVE('',#12141,#12141,#10461,.T.);
#14947=EDGE_CURVE('',#12142,#12142,#10462,.T.);
#14948=EDGE_CURVE('',#12137,#12143,#10463,.T.);
#14949=EDGE_CURVE('',#12143,#12143,#10464,.T.);
#14950=EDGE_CURVE('',#12144,#12144,#10465,.T.);
#14951=EDGE_CURVE('',#12145,#12145,#10466,.T.);
#14952=EDGE_CURVE('',#12146,#12146,#10467,.T.);
#14953=EDGE_CURVE('',#12147,#12147,#10468,.T.);
#14954=EDGE_CURVE('',#12148,#12148,#10469,.T.);
#14955=EDGE_CURVE('',#12149,#12149,#10470,.T.);
#14956=EDGE_CURVE('',#12149,#12150,#10471,.T.);
#14957=EDGE_CURVE('',#12150,#12150,#10472,.T.);
#14958=EDGE_CURVE('',#12150,#12151,#2249,.T.);
#14959=EDGE_CURVE('',#12151,#12151,#10473,.T.);
#14960=EDGE_CURVE('',#12040,#12040,#10474,.T.);
#14961=EDGE_CURVE('',#12040,#12149,#2250,.T.);
#14962=EDGE_CURVE('',#12151,#12152,#10475,.T.);
#14963=EDGE_CURVE('',#12152,#12152,#10476,.T.);
#14964=EDGE_CURVE('',#12152,#12153,#2251,.T.);
#14965=EDGE_CURVE('',#12153,#12154,#10477,.T.);
#14966=EDGE_CURVE('',#12154,#12155,#11179,.T.);
#14967=EDGE_CURVE('',#12156,#12155,#157,.T.);
#14968=EDGE_CURVE('',#12156,#12099,#11180,.T.);
#14969=EDGE_CURVE('',#12095,#12098,#10478,.T.);
#14970=EDGE_CURVE('',#12094,#12157,#11181,.T.);
#14971=EDGE_CURVE('',#12158,#12157,#158,.T.);
#14972=EDGE_CURVE('',#12159,#12158,#10479,.T.);
#14973=EDGE_CURVE('',#12160,#12159,#159,.T.);
#14974=EDGE_CURVE('',#12160,#12161,#11182,.T.);
#14975=EDGE_CURVE('',#12162,#12161,#160,.T.);
#14976=EDGE_CURVE('',#12163,#12162,#10480,.T.);
#14977=EDGE_CURVE('',#12164,#12163,#161,.T.);
#14978=EDGE_CURVE('',#12164,#12165,#11183,.T.);
#14979=EDGE_CURVE('',#12166,#12165,#162,.T.);
#14980=EDGE_CURVE('',#12166,#12167,#11184,.T.);
#14981=EDGE_CURVE('',#12167,#12153,#10481,.T.);
#14982=EDGE_CURVE('',#12162,#12168,#11185,.F.);
#14983=EDGE_CURVE('',#12168,#12169,#10482,.T.);
#14984=EDGE_CURVE('',#12169,#12163,#11186,.F.);
#14985=EDGE_CURVE('',#12169,#12168,#2252,.T.);
#14986=EDGE_CURVE('',#12158,#12170,#11187,.F.);
#14987=EDGE_CURVE('',#12170,#12171,#10483,.T.);
#14988=EDGE_CURVE('',#12171,#12159,#11188,.F.);
#14989=EDGE_CURVE('',#12171,#12170,#2253,.T.);
#14990=EDGE_CURVE('',#12097,#12096,#10484,.T.);
#14991=EDGE_CURVE('',#12172,#12126,#10485,.T.);
#14992=EDGE_CURVE('',#12127,#12173,#10486,.T.);
#14993=EDGE_CURVE('',#12173,#12172,#2254,.T.);
#14994=EDGE_CURVE('',#12133,#12174,#10487,.T.);
#14995=EDGE_CURVE('',#12174,#12173,#10488,.T.);
#14996=EDGE_CURVE('',#12132,#12175,#10489,.T.);
#14997=EDGE_CURVE('',#12175,#12174,#2255,.T.);
#14998=EDGE_CURVE('',#12131,#12176,#10490,.T.);
#14999=EDGE_CURVE('',#12176,#12175,#10491,.T.);
#15000=EDGE_CURVE('',#12130,#12177,#10492,.T.);
#15001=EDGE_CURVE('',#12177,#12176,#2256,.T.);
#15002=EDGE_CURVE('',#12129,#12178,#10493,.T.);
#15003=EDGE_CURVE('',#12178,#12177,#10494,.T.);
#15004=EDGE_CURVE('',#12128,#12179,#10495,.T.);
#15005=EDGE_CURVE('',#12179,#12178,#2257,.T.);
#15006=EDGE_CURVE('',#12172,#12179,#10496,.T.);
#15007=EDGE_CURVE('',#12178,#12038,#2258,.T.);
#15008=EDGE_CURVE('',#12177,#12037,#2259,.T.);
#15009=EDGE_CURVE('',#12179,#12041,#2260,.T.);
#15010=EDGE_CURVE('',#12172,#12042,#2261,.T.);
#15011=EDGE_CURVE('',#12173,#12033,#2262,.T.);
#15012=EDGE_CURVE('',#12113,#12180,#10497,.T.);
#15013=EDGE_CURVE('',#12180,#12180,#10498,.T.);
#15014=EDGE_CURVE('',#12180,#12039,#2263,.T.);
#15015=EDGE_CURVE('',#12040,#12039,#2264,.T.);
#15016=EDGE_CURVE('',#12067,#12181,#10499,.T.);
#15017=EDGE_CURVE('',#12181,#12182,#10500,.T.);
#15018=EDGE_CURVE('',#12182,#12182,#10501,.T.);
#15019=EDGE_CURVE('',#12181,#12183,#10502,.T.);
#15020=EDGE_CURVE('',#12183,#12184,#10503,.T.);
#15021=EDGE_CURVE('',#12184,#12067,#10504,.T.);
#15022=EDGE_CURVE('',#12185,#12183,#2265,.T.);
#15023=EDGE_CURVE('',#12186,#12185,#10505,.T.);
#15024=EDGE_CURVE('',#12184,#12186,#2266,.T.);
#15025=EDGE_CURVE('',#12187,#12181,#2267,.T.);
#15026=EDGE_CURVE('',#12188,#12187,#10506,.T.);
#15027=EDGE_CURVE('',#12183,#12188,#2268,.T.);
#15028=EDGE_CURVE('',#12181,#12081,#2269,.T.);
#15029=EDGE_CURVE('',#12189,#12184,#2270,.T.);
#15030=EDGE_CURVE('',#12068,#12189,#10507,.T.);
#15031=EDGE_CURVE('',#12190,#12190,#10508,.T.);
#15032=EDGE_CURVE('',#12190,#12182,#2271,.T.);
#15033=EDGE_CURVE('',#12116,#12191,#10509,.T.);
#15034=EDGE_CURVE('',#12191,#12192,#10510,.T.);
#15035=EDGE_CURVE('',#12192,#12191,#10511,.T.);
#15036=EDGE_CURVE('',#12193,#12193,#10512,.T.);
#15037=EDGE_CURVE('',#12193,#12192,#2272,.T.);
#15038=EDGE_CURVE('',#12190,#12194,#10513,.T.);
#15039=EDGE_CURVE('',#12194,#12194,#10514,.T.);
#15040=EDGE_CURVE('',#12195,#12196,#10515,.T.);
#15041=EDGE_CURVE('',#12196,#12197,#2273,.T.);
#15042=EDGE_CURVE('',#12197,#12198,#10516,.T.);
#15043=EDGE_CURVE('',#12198,#12195,#2274,.T.);
#15044=EDGE_CURVE('',#12199,#12200,#10517,.T.);
#15045=EDGE_CURVE('',#12200,#12198,#10518,.T.);
#15046=EDGE_CURVE('',#12197,#12199,#10519,.T.);
#15047=EDGE_CURVE('',#12201,#12202,#10520,.T.);
#15048=EDGE_CURVE('',#12202,#12200,#2275,.T.);
#15049=EDGE_CURVE('',#12199,#12201,#2276,.T.);
#15050=EDGE_CURVE('',#12203,#12204,#10521,.T.);
#15051=EDGE_CURVE('',#12204,#12202,#10522,.T.);
#15052=EDGE_CURVE('',#12201,#12203,#10523,.T.);
#15053=EDGE_CURVE('',#12205,#12206,#10524,.T.);
#15054=EDGE_CURVE('',#12206,#12204,#2277,.T.);
#15055=EDGE_CURVE('',#12203,#12205,#2278,.T.);
#15056=EDGE_CURVE('',#12207,#12208,#10525,.T.);
#15057=EDGE_CURVE('',#12208,#12206,#10526,.T.);
#15058=EDGE_CURVE('',#12205,#12207,#10527,.T.);
#15059=EDGE_CURVE('',#12209,#12210,#10528,.T.);
#15060=EDGE_CURVE('',#12210,#12208,#2279,.T.);
#15061=EDGE_CURVE('',#12207,#12209,#2280,.T.);
#15062=EDGE_CURVE('',#12195,#12210,#10529,.T.);
#15063=EDGE_CURVE('',#12209,#12196,#10530,.T.);
#15064=EDGE_CURVE('',#12201,#12211,#2281,.T.);
#15065=EDGE_CURVE('',#12212,#12211,#10531,.T.);
#15066=EDGE_CURVE('',#12203,#12212,#2282,.T.);
#15067=EDGE_CURVE('',#12199,#12213,#2283,.T.);
#15068=EDGE_CURVE('',#12211,#12213,#2284,.T.);
#15069=EDGE_CURVE('',#12197,#12214,#2285,.T.);
#15070=EDGE_CURVE('',#12213,#12214,#10532,.T.);
#15071=EDGE_CURVE('',#12196,#12215,#2286,.T.);
#15072=EDGE_CURVE('',#12214,#12215,#2287,.T.);
#15073=EDGE_CURVE('',#12216,#12217,#2288,.T.);
#15074=EDGE_CURVE('',#12216,#12164,#2289,.T.);
#15075=EDGE_CURVE('',#12217,#12161,#2290,.T.);
#15076=EDGE_CURVE('',#12218,#12214,#10533,.T.);
#15077=EDGE_CURVE('',#12215,#12219,#10534,.T.);
#15078=EDGE_CURVE('',#12219,#12218,#2291,.T.);
#15079=EDGE_CURVE('',#12220,#12221,#10535,.T.);
#15080=EDGE_CURVE('',#12221,#12219,#10536,.T.);
#15081=EDGE_CURVE('',#12215,#12220,#10537,.T.);
#15082=EDGE_CURVE('',#12222,#12223,#10538,.T.);
#15083=EDGE_CURVE('',#12223,#12221,#2292,.T.);
#15084=EDGE_CURVE('',#12220,#12222,#2293,.T.);
#15085=EDGE_CURVE('',#12224,#12225,#10539,.T.);
#15086=EDGE_CURVE('',#12225,#12223,#10540,.T.);
#15087=EDGE_CURVE('',#12222,#12224,#10541,.T.);
#15088=EDGE_CURVE('',#12212,#12226,#10542,.T.);
#15089=EDGE_CURVE('',#12226,#12225,#2294,.T.);
#15090=EDGE_CURVE('',#12224,#12212,#2295,.T.);
#15091=EDGE_CURVE('',#12211,#12227,#10543,.T.);
#15092=EDGE_CURVE('',#12227,#12226,#10544,.T.);
#15093=EDGE_CURVE('',#12213,#12228,#10545,.T.);
#15094=EDGE_CURVE('',#12228,#12227,#2296,.T.);
#15095=EDGE_CURVE('',#12218,#12228,#10546,.T.);
#15096=EDGE_CURVE('',#12205,#12224,#2297,.T.);
#15097=EDGE_CURVE('',#12207,#12222,#2298,.T.);
#15098=EDGE_CURVE('',#12209,#12220,#2299,.T.);
#15099=EDGE_CURVE('',#12028,#12185,#2300,.T.);
#15100=EDGE_CURVE('',#12021,#12188,#2301,.T.);
#15101=EDGE_CURVE('',#12229,#12092,#10547,.T.);
#15102=EDGE_CURVE('',#12093,#12230,#10548,.T.);
#15103=EDGE_CURVE('',#12230,#12229,#2302,.T.);
#15104=EDGE_CURVE('',#12231,#12232,#10549,.T.);
#15105=EDGE_CURVE('',#12232,#12230,#10550,.T.);
#15106=EDGE_CURVE('',#12093,#12231,#10551,.T.);
#15107=EDGE_CURVE('',#12233,#12234,#10552,.T.);
#15108=EDGE_CURVE('',#12234,#12232,#2303,.T.);
#15109=EDGE_CURVE('',#12231,#12233,#2304,.T.);
#15110=EDGE_CURVE('',#12216,#12235,#10553,.T.);
#15111=EDGE_CURVE('',#12235,#12234,#10554,.T.);
#15112=EDGE_CURVE('',#12233,#12216,#10555,.T.);
#15113=EDGE_CURVE('',#12217,#12236,#10556,.T.);
#15114=EDGE_CURVE('',#12236,#12235,#2305,.T.);
#15115=EDGE_CURVE('',#12237,#12238,#10557,.T.);
#15116=EDGE_CURVE('',#12238,#12236,#10558,.T.);
#15117=EDGE_CURVE('',#12217,#12237,#10559,.T.);
#15118=EDGE_CURVE('',#12239,#12240,#10560,.T.);
#15119=EDGE_CURVE('',#12240,#12238,#2306,.T.);
#15120=EDGE_CURVE('',#12237,#12239,#2307,.T.);
#15121=EDGE_CURVE('',#12239,#12092,#10561,.T.);
#15122=EDGE_CURVE('',#12229,#12240,#10562,.T.);
#15123=EDGE_CURVE('',#12233,#12165,#2308,.T.);
#15124=EDGE_CURVE('',#12231,#12156,#2309,.T.);
#15125=EDGE_CURVE('',#12155,#12241,#10563,.T.);
#15126=EDGE_CURVE('',#12241,#12242,#2310,.T.);
#15127=EDGE_CURVE('',#12242,#12243,#10564,.T.);
#15128=EDGE_CURVE('',#12243,#12244,#2311,.T.);
#15129=EDGE_CURVE('',#12244,#12245,#10565,.T.);
#15130=EDGE_CURVE('',#12245,#12246,#2312,.T.);
#15131=EDGE_CURVE('',#12246,#12166,#10566,.T.);
#15132=EDGE_CURVE('',#12247,#12247,#10567,.T.);
#15133=EDGE_CURVE('',#12103,#12248,#10568,.T.);
#15134=EDGE_CURVE('',#12248,#12249,#2313,.T.);
#15135=EDGE_CURVE('',#12249,#12102,#10569,.T.);
#15136=EDGE_CURVE('',#12250,#12104,#10570,.T.);
#15137=EDGE_CURVE('',#12249,#12250,#10571,.T.);
#15138=EDGE_CURVE('',#12251,#12105,#10572,.T.);
#15139=EDGE_CURVE('',#12250,#12251,#2314,.T.);
#15140=EDGE_CURVE('',#12252,#12106,#10573,.T.);
#15141=EDGE_CURVE('',#12251,#12252,#10574,.T.);
#15142=EDGE_CURVE('',#12253,#12107,#10575,.T.);
#15143=EDGE_CURVE('',#12252,#12253,#2315,.T.);
#15144=EDGE_CURVE('',#12254,#12108,#10576,.T.);
#15145=EDGE_CURVE('',#12253,#12254,#10577,.T.);
#15146=EDGE_CURVE('',#12255,#12109,#10578,.T.);
#15147=EDGE_CURVE('',#12254,#12255,#2316,.T.);
#15148=EDGE_CURVE('',#12255,#12248,#10579,.T.);
#15149=EDGE_CURVE('',#12251,#12256,#2317,.T.);
#15150=EDGE_CURVE('',#12257,#12256,#10580,.T.);
#15151=EDGE_CURVE('',#12252,#12257,#2318,.T.);
#15152=EDGE_CURVE('',#12250,#12258,#2319,.T.);
#15153=EDGE_CURVE('',#12256,#12258,#2320,.T.);
#15154=EDGE_CURVE('',#12249,#12259,#2321,.T.);
#15155=EDGE_CURVE('',#12258,#12259,#10581,.T.);
#15156=EDGE_CURVE('',#12248,#12260,#2322,.T.);
#15157=EDGE_CURVE('',#12259,#12260,#2323,.T.);
#15158=EDGE_CURVE('',#12070,#12259,#10582,.T.);
#15159=EDGE_CURVE('',#12260,#12069,#10583,.T.);
#15160=EDGE_CURVE('',#12261,#12071,#10584,.T.);
#15161=EDGE_CURVE('',#12260,#12261,#10585,.T.);
#15162=EDGE_CURVE('',#12262,#12072,#10586,.T.);
#15163=EDGE_CURVE('',#12261,#12262,#2324,.T.);
#15164=EDGE_CURVE('',#12263,#12073,#10587,.T.);
#15165=EDGE_CURVE('',#12262,#12263,#10588,.T.);
#15166=EDGE_CURVE('',#12257,#12074,#10589,.T.);
#15167=EDGE_CURVE('',#12263,#12257,#2325,.T.);
#15168=EDGE_CURVE('',#12256,#12075,#10590,.T.);
#15169=EDGE_CURVE('',#12258,#12076,#10591,.T.);
#15170=EDGE_CURVE('',#12253,#12263,#2326,.T.);
#15171=EDGE_CURVE('',#12254,#12262,#2327,.T.);
#15172=EDGE_CURVE('',#12255,#12261,#2328,.T.);
#15173=EDGE_CURVE('',#12138,#12148,#2329,.T.);
#15174=EDGE_CURVE('',#12139,#12147,#2330,.T.);
#15175=EDGE_CURVE('',#12140,#12146,#2331,.T.);
#15176=EDGE_CURVE('',#12141,#12145,#2332,.T.);
#15177=EDGE_CURVE('',#12264,#12264,#10592,.T.);
#15178=EDGE_CURVE('',#12265,#12265,#10593,.T.);
#15179=EDGE_CURVE('',#12264,#12030,#2333,.T.);
#15180=EDGE_CURVE('',#12266,#12266,#10594,.T.);
#15181=EDGE_CURVE('',#12267,#12267,#10595,.T.);
#15182=EDGE_CURVE('',#12266,#12265,#2334,.T.);
#15183=EDGE_CURVE('',#12027,#12186,#2335,.T.);
#15184=EDGE_CURVE('',#12026,#12189,#2336,.T.);
#15185=EDGE_CURVE('',#12022,#12187,#2337,.T.);
#15186=EDGE_CURVE('',#12176,#12036,#2338,.T.);
#15187=EDGE_CURVE('',#12175,#12035,#2339,.T.);
#15188=EDGE_CURVE('',#12174,#12034,#2340,.T.);
#15189=EDGE_CURVE('',#12044,#12243,#2341,.T.);
#15190=EDGE_CURVE('',#12045,#12244,#2342,.T.);
#15191=EDGE_CURVE('',#12046,#12242,#2343,.T.);
#15192=EDGE_CURVE('',#12047,#12241,#2344,.T.);
#15193=EDGE_CURVE('',#12048,#12154,#2345,.T.);
#15194=EDGE_CURVE('',#12049,#12167,#2346,.T.);
#15195=EDGE_CURVE('',#12050,#12246,#2347,.T.);
#15196=EDGE_CURVE('',#12051,#12245,#2348,.T.);
#15197=EDGE_CURVE('',#12237,#12160,#2349,.T.);
#15198=EDGE_CURVE('',#12239,#12157,#2350,.T.);
#15199=EDGE_CURVE('',#12267,#12144,#2351,.T.);
#15200=EDGE_CURVE('',#12247,#12142,#2352,.T.);
#19556=ORIENTED_EDGE('',*,*,#14782,.T.);
#19557=ORIENTED_EDGE('',*,*,#14783,.T.);
#19558=ORIENTED_EDGE('',*,*,#14784,.T.);
#19559=ORIENTED_EDGE('',*,*,#14783,.F.);
#19560=ORIENTED_EDGE('',*,*,#14785,.F.);
#19561=ORIENTED_EDGE('',*,*,#14786,.T.);
#19562=ORIENTED_EDGE('',*,*,#14784,.F.);
#19563=ORIENTED_EDGE('',*,*,#14786,.F.);
#19564=ORIENTED_EDGE('',*,*,#14787,.T.);
#19565=ORIENTED_EDGE('',*,*,#14788,.F.);
#19566=ORIENTED_EDGE('',*,*,#14789,.T.);
#19567=ORIENTED_EDGE('',*,*,#14790,.F.);
#19568=ORIENTED_EDGE('',*,*,#14791,.T.);
#19569=ORIENTED_EDGE('',*,*,#14792,.F.);
#19570=ORIENTED_EDGE('',*,*,#14793,.T.);
#19571=ORIENTED_EDGE('',*,*,#14794,.F.);
#19572=ORIENTED_EDGE('',*,*,#14782,.F.);
#19573=ORIENTED_EDGE('',*,*,#14785,.T.);
#19574=ORIENTED_EDGE('',*,*,#14795,.T.);
#19575=ORIENTED_EDGE('',*,*,#14796,.T.);
#19576=ORIENTED_EDGE('',*,*,#14795,.F.);
#19577=ORIENTED_EDGE('',*,*,#14797,.F.);
#19578=ORIENTED_EDGE('',*,*,#14796,.F.);
#19579=ORIENTED_EDGE('',*,*,#14798,.T.);
#19580=ORIENTED_EDGE('',*,*,#14799,.T.);
#19581=ORIENTED_EDGE('',*,*,#14800,.T.);
#19582=ORIENTED_EDGE('',*,*,#14799,.F.);
#19583=ORIENTED_EDGE('',*,*,#14801,.T.);
#19584=ORIENTED_EDGE('',*,*,#14802,.T.);
#19585=ORIENTED_EDGE('',*,*,#14803,.T.);
#19586=ORIENTED_EDGE('',*,*,#14804,.T.);
#19587=ORIENTED_EDGE('',*,*,#14805,.T.);
#19588=ORIENTED_EDGE('',*,*,#14806,.T.);
#19589=ORIENTED_EDGE('',*,*,#14807,.F.);
#19590=ORIENTED_EDGE('',*,*,#14807,.T.);
#19591=ORIENTED_EDGE('',*,*,#14808,.T.);
#19592=ORIENTED_EDGE('',*,*,#14809,.T.);
#19593=ORIENTED_EDGE('',*,*,#14810,.T.);
#19594=ORIENTED_EDGE('',*,*,#14811,.F.);
#19595=ORIENTED_EDGE('',*,*,#14812,.F.);
#19596=ORIENTED_EDGE('',*,*,#14813,.F.);
#19597=ORIENTED_EDGE('',*,*,#14814,.F.);
#19598=ORIENTED_EDGE('',*,*,#14815,.F.);
#19599=ORIENTED_EDGE('',*,*,#14816,.F.);
#19600=ORIENTED_EDGE('',*,*,#14817,.F.);
#19601=ORIENTED_EDGE('',*,*,#14818,.F.);
#19602=ORIENTED_EDGE('',*,*,#14819,.F.);
#19603=ORIENTED_EDGE('',*,*,#14798,.F.);
#19604=ORIENTED_EDGE('',*,*,#14800,.F.);
#19605=ORIENTED_EDGE('',*,*,#14820,.T.);
#19606=ORIENTED_EDGE('',*,*,#14821,.F.);
#19607=ORIENTED_EDGE('',*,*,#14820,.F.);
#19608=ORIENTED_EDGE('',*,*,#14811,.T.);
#19609=ORIENTED_EDGE('',*,*,#14822,.T.);
#19610=ORIENTED_EDGE('',*,*,#14823,.T.);
#19611=ORIENTED_EDGE('',*,*,#14822,.F.);
#19612=ORIENTED_EDGE('',*,*,#14823,.F.);
#19613=ORIENTED_EDGE('',*,*,#14824,.T.);
#19614=ORIENTED_EDGE('',*,*,#14825,.F.);
#19615=ORIENTED_EDGE('',*,*,#14824,.F.);
#19616=ORIENTED_EDGE('',*,*,#14826,.T.);
#19617=ORIENTED_EDGE('',*,*,#14827,.T.);
#19618=ORIENTED_EDGE('',*,*,#14828,.T.);
#19619=ORIENTED_EDGE('',*,*,#14829,.T.);
#19620=ORIENTED_EDGE('',*,*,#14826,.F.);
#19621=ORIENTED_EDGE('',*,*,#14830,.T.);
#19622=ORIENTED_EDGE('',*,*,#14828,.F.);
#19623=ORIENTED_EDGE('',*,*,#14831,.T.);
#19624=ORIENTED_EDGE('',*,*,#14832,.T.);
#19625=ORIENTED_EDGE('',*,*,#14829,.F.);
#19626=ORIENTED_EDGE('',*,*,#14833,.F.);
#19627=ORIENTED_EDGE('',*,*,#14834,.F.);
#19628=ORIENTED_EDGE('',*,*,#14835,.F.);
#19629=ORIENTED_EDGE('',*,*,#14790,.T.);
#19630=ORIENTED_EDGE('',*,*,#14836,.T.);
#19631=ORIENTED_EDGE('',*,*,#14837,.F.);
#19632=ORIENTED_EDGE('',*,*,#14838,.T.);
#19633=ORIENTED_EDGE('',*,*,#14839,.F.);
#19634=ORIENTED_EDGE('',*,*,#14840,.T.);
#19635=ORIENTED_EDGE('',*,*,#14841,.T.);
#19636=ORIENTED_EDGE('',*,*,#14842,.T.);
#19637=ORIENTED_EDGE('',*,*,#14843,.F.);
#19638=ORIENTED_EDGE('',*,*,#14844,.F.);
#19639=ORIENTED_EDGE('',*,*,#14845,.F.);
#19640=ORIENTED_EDGE('',*,*,#14846,.F.);
#19641=ORIENTED_EDGE('',*,*,#14847,.F.);
#19642=ORIENTED_EDGE('',*,*,#14848,.F.);
#19643=ORIENTED_EDGE('',*,*,#14849,.F.);
#19644=ORIENTED_EDGE('',*,*,#14850,.F.);
#19645=ORIENTED_EDGE('',*,*,#14851,.F.);
#19646=ORIENTED_EDGE('',*,*,#14852,.F.);
#19647=ORIENTED_EDGE('',*,*,#14853,.T.);
#19648=ORIENTED_EDGE('',*,*,#14831,.F.);
#19649=ORIENTED_EDGE('',*,*,#14827,.F.);
#19650=ORIENTED_EDGE('',*,*,#14832,.F.);
#19651=ORIENTED_EDGE('',*,*,#14853,.F.);
#19652=ORIENTED_EDGE('',*,*,#14854,.T.);
#19653=ORIENTED_EDGE('',*,*,#14855,.T.);
#19654=ORIENTED_EDGE('',*,*,#14856,.T.);
#19655=ORIENTED_EDGE('',*,*,#14857,.T.);
#19656=ORIENTED_EDGE('',*,*,#14837,.T.);
#19657=ORIENTED_EDGE('',*,*,#14854,.F.);
#19658=ORIENTED_EDGE('',*,*,#14858,.T.);
#19659=ORIENTED_EDGE('',*,*,#14857,.F.);
#19660=ORIENTED_EDGE('',*,*,#14859,.T.);
#19661=ORIENTED_EDGE('',*,*,#14858,.F.);
#19662=ORIENTED_EDGE('',*,*,#14836,.F.);
#19663=ORIENTED_EDGE('',*,*,#14789,.F.);
#19664=ORIENTED_EDGE('',*,*,#14860,.T.);
#19665=ORIENTED_EDGE('',*,*,#14861,.T.);
#19666=ORIENTED_EDGE('',*,*,#14840,.F.);
#19667=ORIENTED_EDGE('',*,*,#14862,.F.);
#19668=ORIENTED_EDGE('',*,*,#14838,.F.);
#19669=ORIENTED_EDGE('',*,*,#14863,.F.);
#19670=ORIENTED_EDGE('',*,*,#14864,.T.);
#19671=ORIENTED_EDGE('',*,*,#14855,.F.);
#19672=ORIENTED_EDGE('',*,*,#14859,.F.);
#19673=ORIENTED_EDGE('',*,*,#14856,.F.);
#19674=ORIENTED_EDGE('',*,*,#14864,.F.);
#19675=ORIENTED_EDGE('',*,*,#14865,.T.);
#19676=ORIENTED_EDGE('',*,*,#14866,.T.);
#19677=ORIENTED_EDGE('',*,*,#14867,.T.);
#19678=ORIENTED_EDGE('',*,*,#14834,.T.);
#19679=ORIENTED_EDGE('',*,*,#14865,.F.);
#19680=ORIENTED_EDGE('',*,*,#14868,.T.);
#19681=ORIENTED_EDGE('',*,*,#14867,.F.);
#19682=ORIENTED_EDGE('',*,*,#14869,.T.);
#19683=ORIENTED_EDGE('',*,*,#14870,.T.);
#19684=ORIENTED_EDGE('',*,*,#14871,.F.);
#19685=ORIENTED_EDGE('',*,*,#14872,.T.);
#19686=ORIENTED_EDGE('',*,*,#14869,.F.);
#19687=ORIENTED_EDGE('',*,*,#14866,.F.);
#19688=ORIENTED_EDGE('',*,*,#14870,.F.);
#19689=ORIENTED_EDGE('',*,*,#14872,.F.);
#19690=ORIENTED_EDGE('',*,*,#14873,.T.);
#19691=ORIENTED_EDGE('',*,*,#14874,.T.);
#19692=ORIENTED_EDGE('',*,*,#14875,.T.);
#19693=ORIENTED_EDGE('',*,*,#14876,.T.);
#19694=ORIENTED_EDGE('',*,*,#14839,.T.);
#19695=ORIENTED_EDGE('',*,*,#14873,.F.);
#19696=ORIENTED_EDGE('',*,*,#14862,.T.);
#19697=ORIENTED_EDGE('',*,*,#14876,.F.);
#19698=ORIENTED_EDGE('',*,*,#14877,.T.);
#19699=ORIENTED_EDGE('',*,*,#14878,.F.);
#19700=ORIENTED_EDGE('',*,*,#14879,.T.);
#19701=ORIENTED_EDGE('',*,*,#14874,.F.);
#19702=ORIENTED_EDGE('',*,*,#14877,.F.);
#19703=ORIENTED_EDGE('',*,*,#14875,.F.);
#19704=ORIENTED_EDGE('',*,*,#14879,.F.);
#19705=ORIENTED_EDGE('',*,*,#14880,.T.);
#19706=ORIENTED_EDGE('',*,*,#14881,.T.);
#19707=ORIENTED_EDGE('',*,*,#14878,.T.);
#19708=ORIENTED_EDGE('',*,*,#14881,.F.);
#19709=ORIENTED_EDGE('',*,*,#14882,.F.);
#19710=ORIENTED_EDGE('',*,*,#14883,.T.);
#19711=ORIENTED_EDGE('',*,*,#14884,.T.);
#19712=ORIENTED_EDGE('',*,*,#14885,.F.);
#19713=ORIENTED_EDGE('',*,*,#14886,.T.);
#19714=ORIENTED_EDGE('',*,*,#14887,.F.);
#19715=ORIENTED_EDGE('',*,*,#14888,.T.);
#19716=ORIENTED_EDGE('',*,*,#14889,.F.);
#19717=ORIENTED_EDGE('',*,*,#14890,.F.);
#19718=ORIENTED_EDGE('',*,*,#14891,.F.);
#19719=ORIENTED_EDGE('',*,*,#14892,.F.);
#19720=ORIENTED_EDGE('',*,*,#14893,.F.);
#19721=ORIENTED_EDGE('',*,*,#14894,.F.);
#19722=ORIENTED_EDGE('',*,*,#14895,.F.);
#19723=ORIENTED_EDGE('',*,*,#14896,.F.);
#19724=ORIENTED_EDGE('',*,*,#14897,.F.);
#19725=ORIENTED_EDGE('',*,*,#14898,.F.);
#19726=ORIENTED_EDGE('',*,*,#14899,.F.);
#19727=ORIENTED_EDGE('',*,*,#14900,.F.);
#19728=ORIENTED_EDGE('',*,*,#14880,.F.);
#19729=ORIENTED_EDGE('',*,*,#14890,.T.);
#19730=ORIENTED_EDGE('',*,*,#14901,.T.);
#19731=ORIENTED_EDGE('',*,*,#14871,.T.);
#19732=ORIENTED_EDGE('',*,*,#14901,.F.);
#19733=ORIENTED_EDGE('',*,*,#14900,.T.);
#19734=ORIENTED_EDGE('',*,*,#14902,.T.);
#19735=ORIENTED_EDGE('',*,*,#14863,.T.);
#19736=ORIENTED_EDGE('',*,*,#14902,.F.);
#19737=ORIENTED_EDGE('',*,*,#14891,.T.);
#19738=ORIENTED_EDGE('',*,*,#14903,.T.);
#19739=ORIENTED_EDGE('',*,*,#14852,.T.);
#19740=ORIENTED_EDGE('',*,*,#14903,.F.);
#19741=ORIENTED_EDGE('',*,*,#14904,.T.);
#19742=ORIENTED_EDGE('',*,*,#14905,.T.);
#19743=ORIENTED_EDGE('',*,*,#14906,.T.);
#19744=ORIENTED_EDGE('',*,*,#14905,.F.);
#19745=ORIENTED_EDGE('',*,*,#14907,.F.);
#19746=ORIENTED_EDGE('',*,*,#14908,.F.);
#19747=ORIENTED_EDGE('',*,*,#14909,.F.);
#19748=ORIENTED_EDGE('',*,*,#14910,.F.);
#19749=ORIENTED_EDGE('',*,*,#14911,.F.);
#19750=ORIENTED_EDGE('',*,*,#14904,.F.);
#19751=ORIENTED_EDGE('',*,*,#14912,.F.);
#19752=ORIENTED_EDGE('',*,*,#14913,.T.);
#19753=ORIENTED_EDGE('',*,*,#14906,.F.);
#19754=ORIENTED_EDGE('',*,*,#14913,.F.);
#19755=ORIENTED_EDGE('',*,*,#14908,.T.);
#19756=ORIENTED_EDGE('',*,*,#14914,.T.);
#19757=ORIENTED_EDGE('',*,*,#14915,.T.);
#19758=ORIENTED_EDGE('',*,*,#14914,.F.);
#19759=ORIENTED_EDGE('',*,*,#14916,.F.);
#19760=ORIENTED_EDGE('',*,*,#14917,.T.);
#19761=ORIENTED_EDGE('',*,*,#14915,.F.);
#19762=ORIENTED_EDGE('',*,*,#14917,.F.);
#19763=ORIENTED_EDGE('',*,*,#14911,.T.);
#19764=ORIENTED_EDGE('',*,*,#14918,.T.);
#19765=ORIENTED_EDGE('',*,*,#14919,.T.);
#19766=ORIENTED_EDGE('',*,*,#14918,.F.);
#19767=ORIENTED_EDGE('',*,*,#14920,.F.);
#19768=ORIENTED_EDGE('',*,*,#14921,.T.);
#19769=ORIENTED_EDGE('',*,*,#14919,.F.);
#19770=ORIENTED_EDGE('',*,*,#14921,.F.);
#19771=ORIENTED_EDGE('',*,*,#14909,.T.);
#19772=ORIENTED_EDGE('',*,*,#14922,.T.);
#19773=ORIENTED_EDGE('',*,*,#14923,.T.);
#19774=ORIENTED_EDGE('',*,*,#14922,.F.);
#19775=ORIENTED_EDGE('',*,*,#14924,.F.);
#19776=ORIENTED_EDGE('',*,*,#14925,.T.);
#19777=ORIENTED_EDGE('',*,*,#14923,.F.);
#19778=ORIENTED_EDGE('',*,*,#14925,.F.);
#19779=ORIENTED_EDGE('',*,*,#14926,.T.);
#19780=ORIENTED_EDGE('',*,*,#14927,.T.);
#19781=ORIENTED_EDGE('',*,*,#14825,.T.);
#19782=ORIENTED_EDGE('',*,*,#14927,.F.);
#19783=ORIENTED_EDGE('',*,*,#14928,.F.);
#19784=ORIENTED_EDGE('',*,*,#14929,.F.);
#19785=ORIENTED_EDGE('',*,*,#14930,.F.);
#19786=ORIENTED_EDGE('',*,*,#14931,.F.);
#19787=ORIENTED_EDGE('',*,*,#14932,.F.);
#19788=ORIENTED_EDGE('',*,*,#14933,.F.);
#19789=ORIENTED_EDGE('',*,*,#14934,.F.);
#19790=ORIENTED_EDGE('',*,*,#14935,.F.);
#19791=ORIENTED_EDGE('',*,*,#14936,.F.);
#19792=ORIENTED_EDGE('',*,*,#14926,.F.);
#19793=ORIENTED_EDGE('',*,*,#14936,.T.);
#19794=ORIENTED_EDGE('',*,*,#14937,.T.);
#19795=ORIENTED_EDGE('',*,*,#14821,.T.);
#19796=ORIENTED_EDGE('',*,*,#14937,.F.);
#19797=ORIENTED_EDGE('',*,*,#14938,.T.);
#19798=ORIENTED_EDGE('',*,*,#14939,.T.);
#19799=ORIENTED_EDGE('',*,*,#14940,.T.);
#19800=ORIENTED_EDGE('',*,*,#14939,.F.);
#19801=ORIENTED_EDGE('',*,*,#14938,.F.);
#19802=ORIENTED_EDGE('',*,*,#14941,.T.);
#19803=ORIENTED_EDGE('',*,*,#14942,.F.);
#19804=ORIENTED_EDGE('',*,*,#14941,.F.);
#19805=ORIENTED_EDGE('',*,*,#14940,.F.);
#19806=ORIENTED_EDGE('',*,*,#14943,.T.);
#19807=ORIENTED_EDGE('',*,*,#14944,.T.);
#19808=ORIENTED_EDGE('',*,*,#14945,.T.);
#19809=ORIENTED_EDGE('',*,*,#14946,.T.);
#19810=ORIENTED_EDGE('',*,*,#14947,.F.);
#19811=ORIENTED_EDGE('',*,*,#14942,.T.);
#19812=ORIENTED_EDGE('',*,*,#14948,.T.);
#19813=ORIENTED_EDGE('',*,*,#14949,.T.);
#19814=ORIENTED_EDGE('',*,*,#14948,.F.);
#19815=ORIENTED_EDGE('',*,*,#14949,.F.);
#19816=ORIENTED_EDGE('',*,*,#14950,.T.);
#19817=ORIENTED_EDGE('',*,*,#14951,.T.);
#19818=ORIENTED_EDGE('',*,*,#14952,.T.);
#19819=ORIENTED_EDGE('',*,*,#14953,.T.);
#19820=ORIENTED_EDGE('',*,*,#14954,.T.);
#19821=ORIENTED_EDGE('',*,*,#14955,.T.);
#19822=ORIENTED_EDGE('',*,*,#14956,.T.);
#19823=ORIENTED_EDGE('',*,*,#14957,.T.);
#19824=ORIENTED_EDGE('',*,*,#14956,.F.);
#19825=ORIENTED_EDGE('',*,*,#14957,.F.);
#19826=ORIENTED_EDGE('',*,*,#14958,.T.);
#19827=ORIENTED_EDGE('',*,*,#14959,.F.);
#19828=ORIENTED_EDGE('',*,*,#14958,.F.);
#19829=ORIENTED_EDGE('',*,*,#14960,.F.);
#19830=ORIENTED_EDGE('',*,*,#14961,.T.);
#19831=ORIENTED_EDGE('',*,*,#14955,.F.);
#19832=ORIENTED_EDGE('',*,*,#14961,.F.);
#19833=ORIENTED_EDGE('',*,*,#14959,.T.);
#19834=ORIENTED_EDGE('',*,*,#14962,.T.);
#19835=ORIENTED_EDGE('',*,*,#14963,.T.);
#19836=ORIENTED_EDGE('',*,*,#14962,.F.);
#19837=ORIENTED_EDGE('',*,*,#14963,.F.);
#19838=ORIENTED_EDGE('',*,*,#14964,.T.);
#19839=ORIENTED_EDGE('',*,*,#14965,.T.);
#19840=ORIENTED_EDGE('',*,*,#14966,.T.);
#19841=ORIENTED_EDGE('',*,*,#14967,.F.);
#19842=ORIENTED_EDGE('',*,*,#14968,.T.);
#19843=ORIENTED_EDGE('',*,*,#14888,.F.);
#19844=ORIENTED_EDGE('',*,*,#14969,.F.);
#19845=ORIENTED_EDGE('',*,*,#14884,.F.);
#19846=ORIENTED_EDGE('',*,*,#14970,.T.);
#19847=ORIENTED_EDGE('',*,*,#14971,.F.);
#19848=ORIENTED_EDGE('',*,*,#14972,.F.);
#19849=ORIENTED_EDGE('',*,*,#14973,.F.);
#19850=ORIENTED_EDGE('',*,*,#14974,.T.);
#19851=ORIENTED_EDGE('',*,*,#14975,.F.);
#19852=ORIENTED_EDGE('',*,*,#14976,.F.);
#19853=ORIENTED_EDGE('',*,*,#14977,.F.);
#19854=ORIENTED_EDGE('',*,*,#14978,.T.);
#19855=ORIENTED_EDGE('',*,*,#14979,.F.);
#19856=ORIENTED_EDGE('',*,*,#14980,.T.);
#19857=ORIENTED_EDGE('',*,*,#14981,.T.);
#19858=ORIENTED_EDGE('',*,*,#14964,.F.);
#19859=ORIENTED_EDGE('',*,*,#14982,.T.);
#19860=ORIENTED_EDGE('',*,*,#14983,.T.);
#19861=ORIENTED_EDGE('',*,*,#14984,.T.);
#19862=ORIENTED_EDGE('',*,*,#14976,.T.);
#19863=ORIENTED_EDGE('',*,*,#14983,.F.);
#19864=ORIENTED_EDGE('',*,*,#14985,.F.);
#19865=ORIENTED_EDGE('',*,*,#14986,.T.);
#19866=ORIENTED_EDGE('',*,*,#14987,.T.);
#19867=ORIENTED_EDGE('',*,*,#14988,.T.);
#19868=ORIENTED_EDGE('',*,*,#14972,.T.);
#19869=ORIENTED_EDGE('',*,*,#14987,.F.);
#19870=ORIENTED_EDGE('',*,*,#14989,.F.);
#19871=ORIENTED_EDGE('',*,*,#14887,.T.);
#19872=ORIENTED_EDGE('',*,*,#14990,.T.);
#19873=ORIENTED_EDGE('',*,*,#14885,.T.);
#19874=ORIENTED_EDGE('',*,*,#14969,.T.);
#19875=ORIENTED_EDGE('',*,*,#14990,.F.);
#19876=ORIENTED_EDGE('',*,*,#14886,.F.);
#19877=ORIENTED_EDGE('',*,*,#14991,.T.);
#19878=ORIENTED_EDGE('',*,*,#14928,.T.);
#19879=ORIENTED_EDGE('',*,*,#14992,.T.);
#19880=ORIENTED_EDGE('',*,*,#14993,.T.);
#19881=ORIENTED_EDGE('',*,*,#14994,.T.);
#19882=ORIENTED_EDGE('',*,*,#14995,.T.);
#19883=ORIENTED_EDGE('',*,*,#14992,.F.);
#19884=ORIENTED_EDGE('',*,*,#14935,.T.);
#19885=ORIENTED_EDGE('',*,*,#14996,.T.);
#19886=ORIENTED_EDGE('',*,*,#14997,.T.);
#19887=ORIENTED_EDGE('',*,*,#14994,.F.);
#19888=ORIENTED_EDGE('',*,*,#14934,.T.);
#19889=ORIENTED_EDGE('',*,*,#14998,.T.);
#19890=ORIENTED_EDGE('',*,*,#14999,.T.);
#19891=ORIENTED_EDGE('',*,*,#14996,.F.);
#19892=ORIENTED_EDGE('',*,*,#14933,.T.);
#19893=ORIENTED_EDGE('',*,*,#15000,.T.);
#19894=ORIENTED_EDGE('',*,*,#15001,.T.);
#19895=ORIENTED_EDGE('',*,*,#14998,.F.);
#19896=ORIENTED_EDGE('',*,*,#14932,.T.);
#19897=ORIENTED_EDGE('',*,*,#15002,.T.);
#19898=ORIENTED_EDGE('',*,*,#15003,.T.);
#19899=ORIENTED_EDGE('',*,*,#15000,.F.);
#19900=ORIENTED_EDGE('',*,*,#14931,.T.);
#19901=ORIENTED_EDGE('',*,*,#15004,.T.);
#19902=ORIENTED_EDGE('',*,*,#15005,.T.);
#19903=ORIENTED_EDGE('',*,*,#15002,.F.);
#19904=ORIENTED_EDGE('',*,*,#14930,.T.);
#19905=ORIENTED_EDGE('',*,*,#14991,.F.);
#19906=ORIENTED_EDGE('',*,*,#15006,.T.);
#19907=ORIENTED_EDGE('',*,*,#15004,.F.);
#19908=ORIENTED_EDGE('',*,*,#14929,.T.);
#19909=ORIENTED_EDGE('',*,*,#15003,.F.);
#19910=ORIENTED_EDGE('',*,*,#15007,.T.);
#19911=ORIENTED_EDGE('',*,*,#14805,.F.);
#19912=ORIENTED_EDGE('',*,*,#15008,.F.);
#19913=ORIENTED_EDGE('',*,*,#15005,.F.);
#19914=ORIENTED_EDGE('',*,*,#15009,.T.);
#19915=ORIENTED_EDGE('',*,*,#14808,.F.);
#19916=ORIENTED_EDGE('',*,*,#14806,.F.);
#19917=ORIENTED_EDGE('',*,*,#15007,.F.);
#19918=ORIENTED_EDGE('',*,*,#15006,.F.);
#19919=ORIENTED_EDGE('',*,*,#15010,.T.);
#19920=ORIENTED_EDGE('',*,*,#14809,.F.);
#19921=ORIENTED_EDGE('',*,*,#15009,.F.);
#19922=ORIENTED_EDGE('',*,*,#14993,.F.);
#19923=ORIENTED_EDGE('',*,*,#15011,.T.);
#19924=ORIENTED_EDGE('',*,*,#14810,.F.);
#19925=ORIENTED_EDGE('',*,*,#15010,.F.);
#19926=ORIENTED_EDGE('',*,*,#14907,.T.);
#19927=ORIENTED_EDGE('',*,*,#15012,.T.);
#19928=ORIENTED_EDGE('',*,*,#15013,.T.);
#19929=ORIENTED_EDGE('',*,*,#15012,.F.);
#19930=ORIENTED_EDGE('',*,*,#15013,.F.);
#19931=ORIENTED_EDGE('',*,*,#15014,.T.);
#19932=ORIENTED_EDGE('',*,*,#15015,.F.);
#19933=ORIENTED_EDGE('',*,*,#14960,.T.);
#19934=ORIENTED_EDGE('',*,*,#15015,.T.);
#19935=ORIENTED_EDGE('',*,*,#15014,.F.);
#19936=ORIENTED_EDGE('',*,*,#15016,.T.);
#19937=ORIENTED_EDGE('',*,*,#15017,.T.);
#19938=ORIENTED_EDGE('',*,*,#15018,.T.);
#19939=ORIENTED_EDGE('',*,*,#15017,.F.);
#19940=ORIENTED_EDGE('',*,*,#15019,.T.);
#19941=ORIENTED_EDGE('',*,*,#15020,.T.);
#19942=ORIENTED_EDGE('',*,*,#15021,.T.);
#19943=ORIENTED_EDGE('',*,*,#15020,.F.);
#19944=ORIENTED_EDGE('',*,*,#15022,.F.);
#19945=ORIENTED_EDGE('',*,*,#15023,.F.);
#19946=ORIENTED_EDGE('',*,*,#15024,.F.);
#19947=ORIENTED_EDGE('',*,*,#15019,.F.);
#19948=ORIENTED_EDGE('',*,*,#15025,.F.);
#19949=ORIENTED_EDGE('',*,*,#15026,.F.);
#19950=ORIENTED_EDGE('',*,*,#15027,.F.);
#19951=ORIENTED_EDGE('',*,*,#15016,.F.);
#19952=ORIENTED_EDGE('',*,*,#14841,.F.);
#19953=ORIENTED_EDGE('',*,*,#14861,.F.);
#19954=ORIENTED_EDGE('',*,*,#15028,.F.);
#19955=ORIENTED_EDGE('',*,*,#15021,.F.);
#19956=ORIENTED_EDGE('',*,*,#15029,.F.);
#19957=ORIENTED_EDGE('',*,*,#15030,.F.);
#19958=ORIENTED_EDGE('',*,*,#14842,.F.);
#19959=ORIENTED_EDGE('',*,*,#15031,.F.);
#19960=ORIENTED_EDGE('',*,*,#15032,.T.);
#19961=ORIENTED_EDGE('',*,*,#15018,.F.);
#19962=ORIENTED_EDGE('',*,*,#15032,.F.);
#19963=ORIENTED_EDGE('',*,*,#14910,.T.);
#19964=ORIENTED_EDGE('',*,*,#15033,.T.);
#19965=ORIENTED_EDGE('',*,*,#15034,.T.);
#19966=ORIENTED_EDGE('',*,*,#15035,.T.);
#19967=ORIENTED_EDGE('',*,*,#15033,.F.);
#19968=ORIENTED_EDGE('',*,*,#15036,.F.);
#19969=ORIENTED_EDGE('',*,*,#15037,.T.);
#19970=ORIENTED_EDGE('',*,*,#15034,.F.);
#19971=ORIENTED_EDGE('',*,*,#15035,.F.);
#19972=ORIENTED_EDGE('',*,*,#15037,.F.);
#19973=ORIENTED_EDGE('',*,*,#15031,.T.);
#19974=ORIENTED_EDGE('',*,*,#15038,.T.);
#19975=ORIENTED_EDGE('',*,*,#15039,.T.);
#19976=ORIENTED_EDGE('',*,*,#15038,.F.);
#19977=ORIENTED_EDGE('',*,*,#15036,.T.);
#19978=ORIENTED_EDGE('',*,*,#15039,.F.);
#19979=ORIENTED_EDGE('',*,*,#15040,.T.);
#19980=ORIENTED_EDGE('',*,*,#15041,.T.);
#19981=ORIENTED_EDGE('',*,*,#15042,.T.);
#19982=ORIENTED_EDGE('',*,*,#15043,.T.);
#19983=ORIENTED_EDGE('',*,*,#15044,.T.);
#19984=ORIENTED_EDGE('',*,*,#15045,.T.);
#19985=ORIENTED_EDGE('',*,*,#15042,.F.);
#19986=ORIENTED_EDGE('',*,*,#15046,.T.);
#19987=ORIENTED_EDGE('',*,*,#15047,.T.);
#19988=ORIENTED_EDGE('',*,*,#15048,.T.);
#19989=ORIENTED_EDGE('',*,*,#15044,.F.);
#19990=ORIENTED_EDGE('',*,*,#15049,.T.);
#19991=ORIENTED_EDGE('',*,*,#15050,.T.);
#19992=ORIENTED_EDGE('',*,*,#15051,.T.);
#19993=ORIENTED_EDGE('',*,*,#15047,.F.);
#19994=ORIENTED_EDGE('',*,*,#15052,.T.);
#19995=ORIENTED_EDGE('',*,*,#15053,.T.);
#19996=ORIENTED_EDGE('',*,*,#15054,.T.);
#19997=ORIENTED_EDGE('',*,*,#15050,.F.);
#19998=ORIENTED_EDGE('',*,*,#15055,.T.);
#19999=ORIENTED_EDGE('',*,*,#15056,.T.);
#20000=ORIENTED_EDGE('',*,*,#15057,.T.);
#20001=ORIENTED_EDGE('',*,*,#15053,.F.);
#20002=ORIENTED_EDGE('',*,*,#15058,.T.);
#20003=ORIENTED_EDGE('',*,*,#15059,.T.);
#20004=ORIENTED_EDGE('',*,*,#15060,.T.);
#20005=ORIENTED_EDGE('',*,*,#15056,.F.);
#20006=ORIENTED_EDGE('',*,*,#15061,.T.);
#20007=ORIENTED_EDGE('',*,*,#15040,.F.);
#20008=ORIENTED_EDGE('',*,*,#15062,.T.);
#20009=ORIENTED_EDGE('',*,*,#15059,.F.);
#20010=ORIENTED_EDGE('',*,*,#15063,.T.);
#20011=ORIENTED_EDGE('',*,*,#15052,.F.);
#20012=ORIENTED_EDGE('',*,*,#15064,.T.);
#20013=ORIENTED_EDGE('',*,*,#15065,.F.);
#20014=ORIENTED_EDGE('',*,*,#15066,.F.);
#20015=ORIENTED_EDGE('',*,*,#15049,.F.);
#20016=ORIENTED_EDGE('',*,*,#15067,.T.);
#20017=ORIENTED_EDGE('',*,*,#15068,.F.);
#20018=ORIENTED_EDGE('',*,*,#15064,.F.);
#20019=ORIENTED_EDGE('',*,*,#15046,.F.);
#20020=ORIENTED_EDGE('',*,*,#15069,.T.);
#20021=ORIENTED_EDGE('',*,*,#15070,.F.);
#20022=ORIENTED_EDGE('',*,*,#15067,.F.);
#20023=ORIENTED_EDGE('',*,*,#15041,.F.);
#20024=ORIENTED_EDGE('',*,*,#15071,.T.);
#20025=ORIENTED_EDGE('',*,*,#15072,.F.);
#20026=ORIENTED_EDGE('',*,*,#15069,.F.);
#20027=ORIENTED_EDGE('',*,*,#15073,.F.);
#20028=ORIENTED_EDGE('',*,*,#15074,.T.);
#20029=ORIENTED_EDGE('',*,*,#14977,.T.);
#20030=ORIENTED_EDGE('',*,*,#14984,.F.);
#20031=ORIENTED_EDGE('',*,*,#14985,.T.);
#20032=ORIENTED_EDGE('',*,*,#14982,.F.);
#20033=ORIENTED_EDGE('',*,*,#14975,.T.);
#20034=ORIENTED_EDGE('',*,*,#15075,.F.);
#20035=ORIENTED_EDGE('',*,*,#15043,.F.);
#20036=ORIENTED_EDGE('',*,*,#15045,.F.);
#20037=ORIENTED_EDGE('',*,*,#15048,.F.);
#20038=ORIENTED_EDGE('',*,*,#15051,.F.);
#20039=ORIENTED_EDGE('',*,*,#15054,.F.);
#20040=ORIENTED_EDGE('',*,*,#15057,.F.);
#20041=ORIENTED_EDGE('',*,*,#15060,.F.);
#20042=ORIENTED_EDGE('',*,*,#15062,.F.);
#20043=ORIENTED_EDGE('',*,*,#15076,.T.);
#20044=ORIENTED_EDGE('',*,*,#15072,.T.);
#20045=ORIENTED_EDGE('',*,*,#15077,.T.);
#20046=ORIENTED_EDGE('',*,*,#15078,.T.);
#20047=ORIENTED_EDGE('',*,*,#15079,.T.);
#20048=ORIENTED_EDGE('',*,*,#15080,.T.);
#20049=ORIENTED_EDGE('',*,*,#15077,.F.);
#20050=ORIENTED_EDGE('',*,*,#15081,.T.);
#20051=ORIENTED_EDGE('',*,*,#15082,.T.);
#20052=ORIENTED_EDGE('',*,*,#15083,.T.);
#20053=ORIENTED_EDGE('',*,*,#15079,.F.);
#20054=ORIENTED_EDGE('',*,*,#15084,.T.);
#20055=ORIENTED_EDGE('',*,*,#15085,.T.);
#20056=ORIENTED_EDGE('',*,*,#15086,.T.);
#20057=ORIENTED_EDGE('',*,*,#15082,.F.);
#20058=ORIENTED_EDGE('',*,*,#15087,.T.);
#20059=ORIENTED_EDGE('',*,*,#15088,.T.);
#20060=ORIENTED_EDGE('',*,*,#15089,.T.);
#20061=ORIENTED_EDGE('',*,*,#15085,.F.);
#20062=ORIENTED_EDGE('',*,*,#15090,.T.);
#20063=ORIENTED_EDGE('',*,*,#15091,.T.);
#20064=ORIENTED_EDGE('',*,*,#15092,.T.);
#20065=ORIENTED_EDGE('',*,*,#15088,.F.);
#20066=ORIENTED_EDGE('',*,*,#15065,.T.);
#20067=ORIENTED_EDGE('',*,*,#15093,.T.);
#20068=ORIENTED_EDGE('',*,*,#15094,.T.);
#20069=ORIENTED_EDGE('',*,*,#15091,.F.);
#20070=ORIENTED_EDGE('',*,*,#15068,.T.);
#20071=ORIENTED_EDGE('',*,*,#15076,.F.);
#20072=ORIENTED_EDGE('',*,*,#15095,.T.);
#20073=ORIENTED_EDGE('',*,*,#15093,.F.);
#20074=ORIENTED_EDGE('',*,*,#15070,.T.);
#20075=ORIENTED_EDGE('',*,*,#15058,.F.);
#20076=ORIENTED_EDGE('',*,*,#15096,.T.);
#20077=ORIENTED_EDGE('',*,*,#15087,.F.);
#20078=ORIENTED_EDGE('',*,*,#15097,.F.);
#20079=ORIENTED_EDGE('',*,*,#15061,.F.);
#20080=ORIENTED_EDGE('',*,*,#15097,.T.);
#20081=ORIENTED_EDGE('',*,*,#15084,.F.);
#20082=ORIENTED_EDGE('',*,*,#15098,.F.);
#20083=ORIENTED_EDGE('',*,*,#15063,.F.);
#20084=ORIENTED_EDGE('',*,*,#15098,.T.);
#20085=ORIENTED_EDGE('',*,*,#15081,.F.);
#20086=ORIENTED_EDGE('',*,*,#15071,.F.);
#20087=ORIENTED_EDGE('',*,*,#14794,.T.);
#20088=ORIENTED_EDGE('',*,*,#15099,.T.);
#20089=ORIENTED_EDGE('',*,*,#15022,.T.);
#20090=ORIENTED_EDGE('',*,*,#15027,.T.);
#20091=ORIENTED_EDGE('',*,*,#15100,.F.);
#20092=ORIENTED_EDGE('',*,*,#15078,.F.);
#20093=ORIENTED_EDGE('',*,*,#15080,.F.);
#20094=ORIENTED_EDGE('',*,*,#15083,.F.);
#20095=ORIENTED_EDGE('',*,*,#15086,.F.);
#20096=ORIENTED_EDGE('',*,*,#15089,.F.);
#20097=ORIENTED_EDGE('',*,*,#15092,.F.);
#20098=ORIENTED_EDGE('',*,*,#15094,.F.);
#20099=ORIENTED_EDGE('',*,*,#15095,.F.);
#20100=ORIENTED_EDGE('',*,*,#15101,.T.);
#20101=ORIENTED_EDGE('',*,*,#14882,.T.);
#20102=ORIENTED_EDGE('',*,*,#15102,.T.);
#20103=ORIENTED_EDGE('',*,*,#15103,.T.);
#20104=ORIENTED_EDGE('',*,*,#15104,.T.);
#20105=ORIENTED_EDGE('',*,*,#15105,.T.);
#20106=ORIENTED_EDGE('',*,*,#15102,.F.);
#20107=ORIENTED_EDGE('',*,*,#15106,.T.);
#20108=ORIENTED_EDGE('',*,*,#15107,.T.);
#20109=ORIENTED_EDGE('',*,*,#15108,.T.);
#20110=ORIENTED_EDGE('',*,*,#15104,.F.);
#20111=ORIENTED_EDGE('',*,*,#15109,.T.);
#20112=ORIENTED_EDGE('',*,*,#15110,.T.);
#20113=ORIENTED_EDGE('',*,*,#15111,.T.);
#20114=ORIENTED_EDGE('',*,*,#15107,.F.);
#20115=ORIENTED_EDGE('',*,*,#15112,.T.);
#20116=ORIENTED_EDGE('',*,*,#15113,.T.);
#20117=ORIENTED_EDGE('',*,*,#15114,.T.);
#20118=ORIENTED_EDGE('',*,*,#15110,.F.);
#20119=ORIENTED_EDGE('',*,*,#15073,.T.);
#20120=ORIENTED_EDGE('',*,*,#15115,.T.);
#20121=ORIENTED_EDGE('',*,*,#15116,.T.);
#20122=ORIENTED_EDGE('',*,*,#15113,.F.);
#20123=ORIENTED_EDGE('',*,*,#15117,.T.);
#20124=ORIENTED_EDGE('',*,*,#15118,.T.);
#20125=ORIENTED_EDGE('',*,*,#15119,.T.);
#20126=ORIENTED_EDGE('',*,*,#15115,.F.);
#20127=ORIENTED_EDGE('',*,*,#15120,.T.);
#20128=ORIENTED_EDGE('',*,*,#15118,.F.);
#20129=ORIENTED_EDGE('',*,*,#15121,.T.);
#20130=ORIENTED_EDGE('',*,*,#15101,.F.);
#20131=ORIENTED_EDGE('',*,*,#15122,.T.);
#20132=ORIENTED_EDGE('',*,*,#15112,.F.);
#20133=ORIENTED_EDGE('',*,*,#15123,.T.);
#20134=ORIENTED_EDGE('',*,*,#14978,.F.);
#20135=ORIENTED_EDGE('',*,*,#15074,.F.);
#20136=ORIENTED_EDGE('',*,*,#15109,.F.);
#20137=ORIENTED_EDGE('',*,*,#15124,.T.);
#20138=ORIENTED_EDGE('',*,*,#14967,.T.);
#20139=ORIENTED_EDGE('',*,*,#15125,.T.);
#20140=ORIENTED_EDGE('',*,*,#15126,.T.);
#20141=ORIENTED_EDGE('',*,*,#15127,.T.);
#20142=ORIENTED_EDGE('',*,*,#15128,.T.);
#20143=ORIENTED_EDGE('',*,*,#15129,.T.);
#20144=ORIENTED_EDGE('',*,*,#15130,.T.);
#20145=ORIENTED_EDGE('',*,*,#15131,.T.);
#20146=ORIENTED_EDGE('',*,*,#14979,.T.);
#20147=ORIENTED_EDGE('',*,*,#15123,.F.);
#20148=ORIENTED_EDGE('',*,*,#15106,.F.);
#20149=ORIENTED_EDGE('',*,*,#14889,.T.);
#20150=ORIENTED_EDGE('',*,*,#14968,.F.);
#20151=ORIENTED_EDGE('',*,*,#15124,.F.);
#20152=ORIENTED_EDGE('',*,*,#15103,.F.);
#20153=ORIENTED_EDGE('',*,*,#15105,.F.);
#20154=ORIENTED_EDGE('',*,*,#15108,.F.);
#20155=ORIENTED_EDGE('',*,*,#15111,.F.);
#20156=ORIENTED_EDGE('',*,*,#15114,.F.);
#20157=ORIENTED_EDGE('',*,*,#15116,.F.);
#20158=ORIENTED_EDGE('',*,*,#15119,.F.);
#20159=ORIENTED_EDGE('',*,*,#15122,.F.);
#20160=ORIENTED_EDGE('',*,*,#15132,.F.);
#20161=ORIENTED_EDGE('',*,*,#15133,.T.);
#20162=ORIENTED_EDGE('',*,*,#15134,.T.);
#20163=ORIENTED_EDGE('',*,*,#15135,.T.);
#20164=ORIENTED_EDGE('',*,*,#14892,.T.);
#20165=ORIENTED_EDGE('',*,*,#15136,.T.);
#20166=ORIENTED_EDGE('',*,*,#14893,.T.);
#20167=ORIENTED_EDGE('',*,*,#15135,.F.);
#20168=ORIENTED_EDGE('',*,*,#15137,.T.);
#20169=ORIENTED_EDGE('',*,*,#15138,.T.);
#20170=ORIENTED_EDGE('',*,*,#14894,.T.);
#20171=ORIENTED_EDGE('',*,*,#15136,.F.);
#20172=ORIENTED_EDGE('',*,*,#15139,.T.);
#20173=ORIENTED_EDGE('',*,*,#15140,.T.);
#20174=ORIENTED_EDGE('',*,*,#14895,.T.);
#20175=ORIENTED_EDGE('',*,*,#15138,.F.);
#20176=ORIENTED_EDGE('',*,*,#15141,.T.);
#20177=ORIENTED_EDGE('',*,*,#15142,.T.);
#20178=ORIENTED_EDGE('',*,*,#14896,.T.);
#20179=ORIENTED_EDGE('',*,*,#15140,.F.);
#20180=ORIENTED_EDGE('',*,*,#15143,.T.);
#20181=ORIENTED_EDGE('',*,*,#15144,.T.);
#20182=ORIENTED_EDGE('',*,*,#14897,.T.);
#20183=ORIENTED_EDGE('',*,*,#15142,.F.);
#20184=ORIENTED_EDGE('',*,*,#15145,.T.);
#20185=ORIENTED_EDGE('',*,*,#15146,.T.);
#20186=ORIENTED_EDGE('',*,*,#14898,.T.);
#20187=ORIENTED_EDGE('',*,*,#15144,.F.);
#20188=ORIENTED_EDGE('',*,*,#15147,.T.);
#20189=ORIENTED_EDGE('',*,*,#15133,.F.);
#20190=ORIENTED_EDGE('',*,*,#14899,.T.);
#20191=ORIENTED_EDGE('',*,*,#15146,.F.);
#20192=ORIENTED_EDGE('',*,*,#15148,.T.);
#20193=ORIENTED_EDGE('',*,*,#15141,.F.);
#20194=ORIENTED_EDGE('',*,*,#15149,.T.);
#20195=ORIENTED_EDGE('',*,*,#15150,.F.);
#20196=ORIENTED_EDGE('',*,*,#15151,.F.);
#20197=ORIENTED_EDGE('',*,*,#15139,.F.);
#20198=ORIENTED_EDGE('',*,*,#15152,.T.);
#20199=ORIENTED_EDGE('',*,*,#15153,.F.);
#20200=ORIENTED_EDGE('',*,*,#15149,.F.);
#20201=ORIENTED_EDGE('',*,*,#15137,.F.);
#20202=ORIENTED_EDGE('',*,*,#15154,.T.);
#20203=ORIENTED_EDGE('',*,*,#15155,.F.);
#20204=ORIENTED_EDGE('',*,*,#15152,.F.);
#20205=ORIENTED_EDGE('',*,*,#15134,.F.);
#20206=ORIENTED_EDGE('',*,*,#15156,.T.);
#20207=ORIENTED_EDGE('',*,*,#15157,.F.);
#20208=ORIENTED_EDGE('',*,*,#15154,.F.);
#20209=ORIENTED_EDGE('',*,*,#15158,.T.);
#20210=ORIENTED_EDGE('',*,*,#15157,.T.);
#20211=ORIENTED_EDGE('',*,*,#15159,.T.);
#20212=ORIENTED_EDGE('',*,*,#14844,.T.);
#20213=ORIENTED_EDGE('',*,*,#15160,.T.);
#20214=ORIENTED_EDGE('',*,*,#14845,.T.);
#20215=ORIENTED_EDGE('',*,*,#15159,.F.);
#20216=ORIENTED_EDGE('',*,*,#15161,.T.);
#20217=ORIENTED_EDGE('',*,*,#15162,.T.);
#20218=ORIENTED_EDGE('',*,*,#14846,.T.);
#20219=ORIENTED_EDGE('',*,*,#15160,.F.);
#20220=ORIENTED_EDGE('',*,*,#15163,.T.);
#20221=ORIENTED_EDGE('',*,*,#15164,.T.);
#20222=ORIENTED_EDGE('',*,*,#14847,.T.);
#20223=ORIENTED_EDGE('',*,*,#15162,.F.);
#20224=ORIENTED_EDGE('',*,*,#15165,.T.);
#20225=ORIENTED_EDGE('',*,*,#15166,.T.);
#20226=ORIENTED_EDGE('',*,*,#14848,.T.);
#20227=ORIENTED_EDGE('',*,*,#15164,.F.);
#20228=ORIENTED_EDGE('',*,*,#15167,.T.);
#20229=ORIENTED_EDGE('',*,*,#15168,.T.);
#20230=ORIENTED_EDGE('',*,*,#14849,.T.);
#20231=ORIENTED_EDGE('',*,*,#15166,.F.);
#20232=ORIENTED_EDGE('',*,*,#15150,.T.);
#20233=ORIENTED_EDGE('',*,*,#15169,.T.);
#20234=ORIENTED_EDGE('',*,*,#14850,.T.);
#20235=ORIENTED_EDGE('',*,*,#15168,.F.);
#20236=ORIENTED_EDGE('',*,*,#15153,.T.);
#20237=ORIENTED_EDGE('',*,*,#15158,.F.);
#20238=ORIENTED_EDGE('',*,*,#14851,.T.);
#20239=ORIENTED_EDGE('',*,*,#15169,.F.);
#20240=ORIENTED_EDGE('',*,*,#15155,.T.);
#20241=ORIENTED_EDGE('',*,*,#15145,.F.);
#20242=ORIENTED_EDGE('',*,*,#15170,.T.);
#20243=ORIENTED_EDGE('',*,*,#15165,.F.);
#20244=ORIENTED_EDGE('',*,*,#15171,.F.);
#20245=ORIENTED_EDGE('',*,*,#15147,.F.);
#20246=ORIENTED_EDGE('',*,*,#15171,.T.);
#20247=ORIENTED_EDGE('',*,*,#15163,.F.);
#20248=ORIENTED_EDGE('',*,*,#15172,.F.);
#20249=ORIENTED_EDGE('',*,*,#15148,.F.);
#20250=ORIENTED_EDGE('',*,*,#15172,.T.);
#20251=ORIENTED_EDGE('',*,*,#15161,.F.);
#20252=ORIENTED_EDGE('',*,*,#15156,.F.);
#20253=ORIENTED_EDGE('',*,*,#14912,.T.);
#20254=ORIENTED_EDGE('',*,*,#14916,.T.);
#20255=ORIENTED_EDGE('',*,*,#14920,.T.);
#20256=ORIENTED_EDGE('',*,*,#14924,.T.);
#20257=ORIENTED_EDGE('',*,*,#14943,.F.);
#20258=ORIENTED_EDGE('',*,*,#15173,.T.);
#20259=ORIENTED_EDGE('',*,*,#14954,.F.);
#20260=ORIENTED_EDGE('',*,*,#15173,.F.);
#20261=ORIENTED_EDGE('',*,*,#14944,.F.);
#20262=ORIENTED_EDGE('',*,*,#15174,.T.);
#20263=ORIENTED_EDGE('',*,*,#14953,.F.);
#20264=ORIENTED_EDGE('',*,*,#15174,.F.);
#20265=ORIENTED_EDGE('',*,*,#14945,.F.);
#20266=ORIENTED_EDGE('',*,*,#15175,.T.);
#20267=ORIENTED_EDGE('',*,*,#14952,.F.);
#20268=ORIENTED_EDGE('',*,*,#15175,.F.);
#20269=ORIENTED_EDGE('',*,*,#14946,.F.);
#20270=ORIENTED_EDGE('',*,*,#15176,.T.);
#20271=ORIENTED_EDGE('',*,*,#14951,.F.);
#20272=ORIENTED_EDGE('',*,*,#15176,.F.);
#20273=ORIENTED_EDGE('',*,*,#15143,.F.);
#20274=ORIENTED_EDGE('',*,*,#15151,.T.);
#20275=ORIENTED_EDGE('',*,*,#15167,.F.);
#20276=ORIENTED_EDGE('',*,*,#15170,.F.);
#20277=ORIENTED_EDGE('',*,*,#15055,.F.);
#20278=ORIENTED_EDGE('',*,*,#15066,.T.);
#20279=ORIENTED_EDGE('',*,*,#15090,.F.);
#20280=ORIENTED_EDGE('',*,*,#15096,.F.);
#20281=ORIENTED_EDGE('',*,*,#15177,.T.);
#20282=ORIENTED_EDGE('',*,*,#15178,.F.);
#20283=ORIENTED_EDGE('',*,*,#15177,.F.);
#20284=ORIENTED_EDGE('',*,*,#15179,.T.);
#20285=ORIENTED_EDGE('',*,*,#14797,.T.);
#20286=ORIENTED_EDGE('',*,*,#15179,.F.);
#20287=ORIENTED_EDGE('',*,*,#15180,.T.);
#20288=ORIENTED_EDGE('',*,*,#15181,.F.);
#20289=ORIENTED_EDGE('',*,*,#15180,.F.);
#20290=ORIENTED_EDGE('',*,*,#15182,.T.);
#20291=ORIENTED_EDGE('',*,*,#15178,.T.);
#20292=ORIENTED_EDGE('',*,*,#15182,.F.);
#20293=ORIENTED_EDGE('',*,*,#14793,.F.);
#20294=ORIENTED_EDGE('',*,*,#15183,.T.);
#20295=ORIENTED_EDGE('',*,*,#15023,.T.);
#20296=ORIENTED_EDGE('',*,*,#15099,.F.);
#20297=ORIENTED_EDGE('',*,*,#14792,.T.);
#20298=ORIENTED_EDGE('',*,*,#15184,.T.);
#20299=ORIENTED_EDGE('',*,*,#15029,.T.);
#20300=ORIENTED_EDGE('',*,*,#15024,.T.);
#20301=ORIENTED_EDGE('',*,*,#15183,.F.);
#20302=ORIENTED_EDGE('',*,*,#14830,.F.);
#20303=ORIENTED_EDGE('',*,*,#14843,.T.);
#20304=ORIENTED_EDGE('',*,*,#15030,.T.);
#20305=ORIENTED_EDGE('',*,*,#15184,.F.);
#20306=ORIENTED_EDGE('',*,*,#14791,.F.);
#20307=ORIENTED_EDGE('',*,*,#14835,.T.);
#20308=ORIENTED_EDGE('',*,*,#14868,.F.);
#20309=ORIENTED_EDGE('',*,*,#14833,.T.);
#20310=ORIENTED_EDGE('',*,*,#14788,.T.);
#20311=ORIENTED_EDGE('',*,*,#15185,.T.);
#20312=ORIENTED_EDGE('',*,*,#15025,.T.);
#20313=ORIENTED_EDGE('',*,*,#15028,.T.);
#20314=ORIENTED_EDGE('',*,*,#14860,.F.);
#20315=ORIENTED_EDGE('',*,*,#14787,.F.);
#20316=ORIENTED_EDGE('',*,*,#15100,.T.);
#20317=ORIENTED_EDGE('',*,*,#15026,.T.);
#20318=ORIENTED_EDGE('',*,*,#15185,.F.);
#20319=ORIENTED_EDGE('',*,*,#15001,.F.);
#20320=ORIENTED_EDGE('',*,*,#15008,.T.);
#20321=ORIENTED_EDGE('',*,*,#14804,.F.);
#20322=ORIENTED_EDGE('',*,*,#15186,.F.);
#20323=ORIENTED_EDGE('',*,*,#14999,.F.);
#20324=ORIENTED_EDGE('',*,*,#15186,.T.);
#20325=ORIENTED_EDGE('',*,*,#14803,.F.);
#20326=ORIENTED_EDGE('',*,*,#15187,.F.);
#20327=ORIENTED_EDGE('',*,*,#14997,.F.);
#20328=ORIENTED_EDGE('',*,*,#15187,.T.);
#20329=ORIENTED_EDGE('',*,*,#14802,.F.);
#20330=ORIENTED_EDGE('',*,*,#15188,.F.);
#20331=ORIENTED_EDGE('',*,*,#14995,.F.);
#20332=ORIENTED_EDGE('',*,*,#15188,.T.);
#20333=ORIENTED_EDGE('',*,*,#14801,.F.);
#20334=ORIENTED_EDGE('',*,*,#15011,.F.);
#20335=ORIENTED_EDGE('',*,*,#15128,.F.);
#20336=ORIENTED_EDGE('',*,*,#15189,.F.);
#20337=ORIENTED_EDGE('',*,*,#14812,.T.);
#20338=ORIENTED_EDGE('',*,*,#15190,.T.);
#20339=ORIENTED_EDGE('',*,*,#15127,.F.);
#20340=ORIENTED_EDGE('',*,*,#15191,.F.);
#20341=ORIENTED_EDGE('',*,*,#14813,.T.);
#20342=ORIENTED_EDGE('',*,*,#15189,.T.);
#20343=ORIENTED_EDGE('',*,*,#15126,.F.);
#20344=ORIENTED_EDGE('',*,*,#15192,.F.);
#20345=ORIENTED_EDGE('',*,*,#14814,.T.);
#20346=ORIENTED_EDGE('',*,*,#15191,.T.);
#20347=ORIENTED_EDGE('',*,*,#15125,.F.);
#20348=ORIENTED_EDGE('',*,*,#14966,.F.);
#20349=ORIENTED_EDGE('',*,*,#15193,.F.);
#20350=ORIENTED_EDGE('',*,*,#14815,.T.);
#20351=ORIENTED_EDGE('',*,*,#15192,.T.);
#20352=ORIENTED_EDGE('',*,*,#14981,.F.);
#20353=ORIENTED_EDGE('',*,*,#15194,.F.);
#20354=ORIENTED_EDGE('',*,*,#14816,.T.);
#20355=ORIENTED_EDGE('',*,*,#15193,.T.);
#20356=ORIENTED_EDGE('',*,*,#14965,.F.);
#20357=ORIENTED_EDGE('',*,*,#15131,.F.);
#20358=ORIENTED_EDGE('',*,*,#15195,.F.);
#20359=ORIENTED_EDGE('',*,*,#14817,.T.);
#20360=ORIENTED_EDGE('',*,*,#15194,.T.);
#20361=ORIENTED_EDGE('',*,*,#14980,.F.);
#20362=ORIENTED_EDGE('',*,*,#15130,.F.);
#20363=ORIENTED_EDGE('',*,*,#15196,.F.);
#20364=ORIENTED_EDGE('',*,*,#14818,.T.);
#20365=ORIENTED_EDGE('',*,*,#15195,.T.);
#20366=ORIENTED_EDGE('',*,*,#15129,.F.);
#20367=ORIENTED_EDGE('',*,*,#15190,.F.);
#20368=ORIENTED_EDGE('',*,*,#14819,.T.);
#20369=ORIENTED_EDGE('',*,*,#15196,.T.);
#20370=ORIENTED_EDGE('',*,*,#15120,.F.);
#20371=ORIENTED_EDGE('',*,*,#15197,.T.);
#20372=ORIENTED_EDGE('',*,*,#14973,.T.);
#20373=ORIENTED_EDGE('',*,*,#14988,.F.);
#20374=ORIENTED_EDGE('',*,*,#14989,.T.);
#20375=ORIENTED_EDGE('',*,*,#14986,.F.);
#20376=ORIENTED_EDGE('',*,*,#14971,.T.);
#20377=ORIENTED_EDGE('',*,*,#15198,.F.);
#20378=ORIENTED_EDGE('',*,*,#15121,.F.);
#20379=ORIENTED_EDGE('',*,*,#15198,.T.);
#20380=ORIENTED_EDGE('',*,*,#14970,.F.);
#20381=ORIENTED_EDGE('',*,*,#14883,.F.);
#20382=ORIENTED_EDGE('',*,*,#15117,.F.);
#20383=ORIENTED_EDGE('',*,*,#15075,.T.);
#20384=ORIENTED_EDGE('',*,*,#14974,.F.);
#20385=ORIENTED_EDGE('',*,*,#15197,.F.);
#20386=ORIENTED_EDGE('',*,*,#15181,.T.);
#20387=ORIENTED_EDGE('',*,*,#15199,.T.);
#20388=ORIENTED_EDGE('',*,*,#14950,.F.);
#20389=ORIENTED_EDGE('',*,*,#15199,.F.);
#20390=ORIENTED_EDGE('',*,*,#15132,.T.);
#20391=ORIENTED_EDGE('',*,*,#15200,.T.);
#20392=ORIENTED_EDGE('',*,*,#14947,.T.);
#20393=ORIENTED_EDGE('',*,*,#15200,.F.);
#25619=TOROIDAL_SURFACE('',#28097,68.,2.);
#25620=TOROIDAL_SURFACE('',#28109,68.,2.);
#25621=TOROIDAL_SURFACE('',#28118,123.013975850864,2.);
#25622=TOROIDAL_SURFACE('',#28126,118.739209725433,2.);
#25623=TOROIDAL_SURFACE('',#28135,63.9364279314891,2.);
#25624=TOROIDAL_SURFACE('',#28138,63.9364279314891,2.);
#25625=TOROIDAL_SURFACE('',#28141,63.9364279314891,2.);
#25626=TOROIDAL_SURFACE('',#28164,123.,2.);
#25627=TOROIDAL_SURFACE('',#28168,47.,2.);
#25628=TOROIDAL_SURFACE('',#28184,92.1,2.);
#25629=TOROIDAL_SURFACE('',#28190,47.,2.);
#25630=TOROIDAL_SURFACE('',#28197,7.99999999999998,2.);
#25631=TOROIDAL_SURFACE('',#28203,7.99999999999999,2.);
#25632=TOROIDAL_SURFACE('',#28209,8.00000000000001,2.);
#25633=TOROIDAL_SURFACE('',#28215,8.00000000000001,2.);
#25634=TOROIDAL_SURFACE('',#28228,8.00000000000001,2.);
#25635=TOROIDAL_SURFACE('',#28234,8.00000000000001,2.);
#25636=TOROIDAL_SURFACE('',#28240,7.99999999999999,2.);
#25637=TOROIDAL_SURFACE('',#28245,7.99999999999998,2.);
#25638=TOROIDAL_SURFACE('',#28254,6.,2.);
#25639=TOROIDAL_SURFACE('',#28260,6.,2.);
#25640=TOROIDAL_SURFACE('',#28266,6.,2.);
#25641=TOROIDAL_SURFACE('',#28272,6.,2.);
#25642=TOROIDAL_SURFACE('',#28287,7.99999999999998,2.);
#25643=TOROIDAL_SURFACE('',#28292,8.00000000000001,2.);
#25644=TOROIDAL_SURFACE('',#28297,8.00000000000001,2.);
#25645=TOROIDAL_SURFACE('',#28302,7.99999999999999,2.);
#25646=TOROIDAL_SURFACE('',#28313,7.99999999999999,2.);
#25647=TOROIDAL_SURFACE('',#28318,8.00000000000001,2.);
#25648=TOROIDAL_SURFACE('',#28323,8.00000000000001,2.);
#25649=TOROIDAL_SURFACE('',#28327,7.99999999999998,2.);
#25996=ADVANCED_FACE('',(#7172),#341,.F.);
#25997=ADVANCED_FACE('',(#7173),#6602,.F.);
#25998=ADVANCED_FACE('',(#7174,#647),#883,.T.);
#25999=ADVANCED_FACE('',(#7175),#342,.F.);
#26000=ADVANCED_FACE('',(#7176,#648),#884,.F.);
#26001=ADVANCED_FACE('',(#7177),#343,.F.);
#26002=ADVANCED_FACE('',(#7178,#649,#650,#651),#885,.T.);
#26003=ADVANCED_FACE('',(#7179),#6603,.F.);
#26004=ADVANCED_FACE('',(#7180),#344,.F.);
#26005=ADVANCED_FACE('',(#7181),#6604,.F.);
#26006=ADVANCED_FACE('',(#7182),#345,.F.);
#26007=ADVANCED_FACE('',(#7183),#567,.T.);
#26008=ADVANCED_FACE('',(#7184,#652),#886,.F.);
#26009=ADVANCED_FACE('',(#7185),#6605,.F.);
#26010=ADVANCED_FACE('',(#7186),#346,.F.);
#26011=ADVANCED_FACE('',(#7187),#568,.T.);
#26012=ADVANCED_FACE('',(#7188),#6606,.F.);
#26013=ADVANCED_FACE('',(#7189),#6607,.F.);
#26014=ADVANCED_FACE('',(#7190),#347,.F.);
#26015=ADVANCED_FACE('',(#7191),#569,.T.);
#26016=ADVANCED_FACE('',(#7192),#6608,.F.);
#26017=ADVANCED_FACE('',(#7193),#348,.F.);
#26018=ADVANCED_FACE('',(#7194),#570,.T.);
#26019=ADVANCED_FACE('',(#7195),#6609,.F.);
#26020=ADVANCED_FACE('',(#7196),#349,.F.);
#26021=ADVANCED_FACE('',(#7197,#653,#654,#655,#656,#657),#887,.T.);
#26022=ADVANCED_FACE('',(#7198),#350,.F.);
#26023=ADVANCED_FACE('',(#7199),#351,.F.);
#26024=ADVANCED_FACE('',(#7200),#352,.F.);
#26025=ADVANCED_FACE('',(#7201),#353,.F.);
#26026=ADVANCED_FACE('',(#7202,#658,#659,#660,#661,#662),#888,.T.);
#26027=ADVANCED_FACE('',(#7203),#6610,.F.);
#26028=ADVANCED_FACE('',(#7204),#354,.F.);
#26029=ADVANCED_FACE('',(#7205),#6611,.F.);
#26030=ADVANCED_FACE('',(#7206),#355,.F.);
#26031=ADVANCED_FACE('',(#7207),#6612,.F.);
#26032=ADVANCED_FACE('',(#7208),#356,.F.);
#26033=ADVANCED_FACE('',(#7209),#6613,.F.);
#26034=ADVANCED_FACE('',(#7210),#357,.F.);
#26035=ADVANCED_FACE('',(#7211,#663,#664),#889,.F.);
#26036=ADVANCED_FACE('',(#7212),#358,.F.);
#26037=ADVANCED_FACE('',(#7213),#25619,.T.);
#26038=ADVANCED_FACE('',(#7214),#6614,.T.);
#26039=ADVANCED_FACE('',(#7215,#665,#666,#667,#668,#669),#890,.T.);
#26040=ADVANCED_FACE('',(#7216),#25620,.T.);
#26041=ADVANCED_FACE('',(#7217,#670,#671,#672,#673,#674),#891,.T.);
#26042=ADVANCED_FACE('',(#7218),#25621,.T.);
#26043=ADVANCED_FACE('',(#7219),#359,.T.);
#26044=ADVANCED_FACE('',(#7220),#360,.T.);
#26045=ADVANCED_FACE('',(#7221),#25622,.T.);
#26046=ADVANCED_FACE('',(#7222),#361,.T.);
#26047=ADVANCED_FACE('',(#7223),#25623,.T.);
#26048=ADVANCED_FACE('',(#7224),#892,.T.);
#26049=ADVANCED_FACE('',(#7225),#25624,.T.);
#26050=ADVANCED_FACE('',(#7226),#893,.T.);
#26051=ADVANCED_FACE('',(#7227),#25625,.T.);
#26052=ADVANCED_FACE('',(#7228),#894,.T.);
#26053=ADVANCED_FACE('',(#7229),#6615,.T.);
#26054=ADVANCED_FACE('',(#7230),#600,.F.);
#26055=ADVANCED_FACE('',(#7231),#6616,.T.);
#26056=ADVANCED_FACE('',(#7232),#601,.F.);
#26057=ADVANCED_FACE('',(#7233),#6617,.T.);
#26058=ADVANCED_FACE('',(#7234),#602,.F.);
#26059=ADVANCED_FACE('',(#7235),#6618,.T.);
#26060=ADVANCED_FACE('',(#7236),#603,.F.);
#26061=ADVANCED_FACE('',(#7237),#6619,.T.);
#26062=ADVANCED_FACE('',(#7238),#895,.T.);
#26063=ADVANCED_FACE('',(#7239),#6620,.T.);
#26064=ADVANCED_FACE('',(#7240),#896,.T.);
#26065=ADVANCED_FACE('',(#7241),#25626,.T.);
#26066=ADVANCED_FACE('',(#7242),#6621,.T.);
#26067=ADVANCED_FACE('',(#7243),#25627,.T.);
#26068=ADVANCED_FACE('',(#7244),#897,.F.);
#26069=ADVANCED_FACE('',(#7245),#898,.F.);
#26070=ADVANCED_FACE('',(#7246),#899,.F.);
#26071=ADVANCED_FACE('',(#7247),#900,.F.);
#26072=ADVANCED_FACE('',(#7248),#6622,.F.);
#26073=ADVANCED_FACE('',(#7249),#25628,.T.);
#26074=ADVANCED_FACE('',(#7250),#6623,.F.);
#26075=ADVANCED_FACE('',(#7251),#25629,.T.);
#26076=ADVANCED_FACE('',(#7252,#675),#901,.F.);
#26077=ADVANCED_FACE('',(#7253),#6624,.T.);
#26078=ADVANCED_FACE('',(#7254),#25630,.T.);
#26079=ADVANCED_FACE('',(#7255),#6625,.T.);
#26080=ADVANCED_FACE('',(#7256),#25631,.T.);
#26081=ADVANCED_FACE('',(#7257),#6626,.T.);
#26082=ADVANCED_FACE('',(#7258),#25632,.T.);
#26083=ADVANCED_FACE('',(#7259),#6627,.T.);
#26084=ADVANCED_FACE('',(#7260),#25633,.T.);
#26085=ADVANCED_FACE('',(#7261),#6628,.F.);
#26086=ADVANCED_FACE('',(#7262),#902,.F.);
#26087=ADVANCED_FACE('',(#7263),#6629,.F.);
#26088=ADVANCED_FACE('',(#7264),#903,.F.);
#26089=ADVANCED_FACE('',(#7265,#676),#904,.T.);
#26090=ADVANCED_FACE('',(#7266),#6630,.T.);
#26091=ADVANCED_FACE('',(#7267),#25634,.T.);
#26092=ADVANCED_FACE('',(#7268),#6631,.T.);
#26093=ADVANCED_FACE('',(#7269),#25635,.T.);
#26094=ADVANCED_FACE('',(#7270),#6632,.T.);
#26095=ADVANCED_FACE('',(#7271),#25636,.T.);
#26096=ADVANCED_FACE('',(#7272),#6633,.T.);
#26097=ADVANCED_FACE('',(#7273),#25637,.T.);
#26098=ADVANCED_FACE('',(#7274),#6634,.F.);
#26099=ADVANCED_FACE('',(#7275),#905,.F.);
#26100=ADVANCED_FACE('',(#7276),#6635,.F.);
#26101=ADVANCED_FACE('',(#7277,#677),#906,.F.);
#26102=ADVANCED_FACE('',(#7278),#6636,.T.);
#26103=ADVANCED_FACE('',(#7279),#25638,.T.);
#26104=ADVANCED_FACE('',(#7280),#6637,.T.);
#26105=ADVANCED_FACE('',(#7281),#25639,.T.);
#26106=ADVANCED_FACE('',(#7282),#6638,.T.);
#26107=ADVANCED_FACE('',(#7283),#25640,.T.);
#26108=ADVANCED_FACE('',(#7284),#6639,.T.);
#26109=ADVANCED_FACE('',(#7285),#25641,.T.);
#26110=ADVANCED_FACE('',(#7286),#6640,.T.);
#26111=ADVANCED_FACE('',(#7287),#907,.T.);
#26112=ADVANCED_FACE('',(#7288),#6641,.T.);
#26113=ADVANCED_FACE('',(#7289,#678),#908,.F.);
#26114=ADVANCED_FACE('',(#7290),#6642,.T.);
#26115=ADVANCED_FACE('',(#7291),#25642,.T.);
#26116=ADVANCED_FACE('',(#7292),#6643,.T.);
#26117=ADVANCED_FACE('',(#7293),#25643,.T.);
#26118=ADVANCED_FACE('',(#7294),#6644,.T.);
#26119=ADVANCED_FACE('',(#7295),#25644,.T.);
#26120=ADVANCED_FACE('',(#7296),#6645,.T.);
#26121=ADVANCED_FACE('',(#7297),#25645,.T.);
#26122=ADVANCED_FACE('',(#7298),#6646,.F.);
#26123=ADVANCED_FACE('',(#7299),#909,.F.);
#26124=ADVANCED_FACE('',(#7300),#6647,.F.);
#26125=ADVANCED_FACE('',(#7301),#910,.F.);
#26126=ADVANCED_FACE('',(#7302),#6648,.T.);
#26127=ADVANCED_FACE('',(#7303),#25646,.T.);
#26128=ADVANCED_FACE('',(#7304),#6649,.T.);
#26129=ADVANCED_FACE('',(#7305),#25647,.T.);
#26130=ADVANCED_FACE('',(#7306),#6650,.T.);
#26131=ADVANCED_FACE('',(#7307),#25648,.T.);
#26132=ADVANCED_FACE('',(#7308),#6651,.T.);
#26133=ADVANCED_FACE('',(#7309),#25649,.T.);
#26134=ADVANCED_FACE('',(#7310),#6652,.F.);
#26135=ADVANCED_FACE('',(#7311),#911,.F.);
#26136=ADVANCED_FACE('',(#7312),#6653,.F.);
#26137=ADVANCED_FACE('',(#7313),#912,.T.);
#26138=ADVANCED_FACE('',(#7314),#913,.T.);
#26139=ADVANCED_FACE('',(#7315),#914,.T.);
#26140=ADVANCED_FACE('',(#7316),#915,.T.);
#26141=ADVANCED_FACE('',(#7317),#6654,.F.);
#26142=ADVANCED_FACE('',(#7318),#6655,.F.);
#26143=ADVANCED_FACE('',(#7319),#6656,.F.);
#26144=ADVANCED_FACE('',(#7320),#6657,.F.);
#26145=ADVANCED_FACE('',(#7321),#916,.F.);
#26146=ADVANCED_FACE('',(#7322),#917,.F.);
#26147=ADVANCED_FACE('',(#7323,#679),#918,.F.);
#26148=ADVANCED_FACE('',(#7324),#6658,.F.);
#26149=ADVANCED_FACE('',(#7325,#680),#919,.F.);
#26150=ADVANCED_FACE('',(#7326),#6659,.F.);
#26151=ADVANCED_FACE('',(#7327),#6660,.F.);
#26152=ADVANCED_FACE('',(#7328),#920,.F.);
#26153=ADVANCED_FACE('',(#7329),#6661,.F.);
#26154=ADVANCED_FACE('',(#7330),#921,.F.);
#26155=ADVANCED_FACE('',(#7331),#6662,.F.);
#26156=ADVANCED_FACE('',(#7332),#922,.T.);
#26157=ADVANCED_FACE('',(#7333),#6663,.T.);
#26158=ADVANCED_FACE('',(#7334),#923,.T.);
#26159=ADVANCED_FACE('',(#7335),#6664,.T.);
#26160=ADVANCED_FACE('',(#7336),#924,.T.);
#26161=ADVANCED_FACE('',(#7337),#6665,.T.);
#26162=ADVANCED_FACE('',(#7338),#925,.T.);
#26163=ADVANCED_FACE('',(#7339),#6666,.T.);
#26164=ADVANCED_FACE('',(#7340),#926,.T.);
#26165=ADVANCED_FACE('',(#7341),#6667,.T.);
#26166=ADVANCED_FACE('',(#7342),#927,.T.);
#26167=ADVANCED_FACE('',(#7343),#6668,.T.);
#26168=ADVANCED_FACE('',(#7344),#928,.T.);
#26169=ADVANCED_FACE('',(#7345),#6669,.T.);
#26170=ADVANCED_FACE('',(#7346),#6670,.T.);
#26171=ADVANCED_FACE('',(#7347),#6671,.F.);
#26172=ADVANCED_FACE('',(#7348),#362,.T.);
#27223=CLOSED_SHELL('',(#25996,#25997,#25998,#25999,#26000,#26001,#26002,
#26003,#26004,#26005,#26006,#26007,#26008,#26009,#26010,#26011,#26012,#26013,
#26014,#26015,#26016,#26017,#26018,#26019,#26020,#26021,#26022,#26023,#26024,
#26025,#26026,#26027,#26028,#26029,#26030,#26031,#26032,#26033,#26034,#26035,
#26036,#26037,#26038,#26039,#26040,#26041,#26042,#26043,#26044,#26045,#26046,
#26047,#26048,#26049,#26050,#26051,#26052,#26053,#26054,#26055,#26056,#26057,
#26058,#26059,#26060,#26061,#26062,#26063,#26064,#26065,#26066,#26067,#26068,
#26069,#26070,#26071,#26072,#26073,#26074,#26075,#26076,#26077,#26078,#26079,
#26080,#26081,#26082,#26083,#26084,#26085,#26086,#26087,#26088,#26089,#26090,
#26091,#26092,#26093,#26094,#26095,#26096,#26097,#26098,#26099,#26100,#26101,
#26102,#26103,#26104,#26105,#26106,#26107,#26108,#26109,#26110,#26111,#26112,
#26113,#26114,#26115,#26116,#26117,#26118,#26119,#26120,#26121,#26122,#26123,
#26124,#26125,#26126,#26127,#26128,#26129,#26130,#26131,#26132,#26133,#26134,
#26135,#26136,#26137,#26138,#26139,#26140,#26141,#26142,#26143,#26144,#26145,
#26146,#26147,#26148,#26149,#26150,#26151,#26152,#26153,#26154,#26155,#26156,
#26157,#26158,#26159,#26160,#26161,#26162,#26163,#26164,#26165,#26166,#26167,
#26168,#26169,#26170,#26171,#26172));
#27989=AXIS2_PLACEMENT_3D('',#41492,#31448,#31449);
#27990=AXIS2_PLACEMENT_3D('',#41493,#31450,#31451);
#27991=AXIS2_PLACEMENT_3D('',#41495,#31452,#31453);
#27992=AXIS2_PLACEMENT_3D('',#41498,#31455,#31456);
#27993=AXIS2_PLACEMENT_3D('',#41499,#31457,#31458);
#27994=AXIS2_PLACEMENT_3D('',#41501,#31459,#31460);
#27995=AXIS2_PLACEMENT_3D('',#41503,#31462,#31463);
#27996=AXIS2_PLACEMENT_3D('',#41506,#31464,#31465);
#27997=AXIS2_PLACEMENT_3D('',#41510,#31467,#31468);
#27998=AXIS2_PLACEMENT_3D('',#41514,#31470,#31471);
#27999=AXIS2_PLACEMENT_3D('',#41518,#31473,#31474);
#28000=AXIS2_PLACEMENT_3D('',#41520,#31476,#31477);
#28001=AXIS2_PLACEMENT_3D('',#41523,#31479,#31480);
#28002=AXIS2_PLACEMENT_3D('',#41524,#31481,#31482);
#28003=AXIS2_PLACEMENT_3D('',#41526,#31483,#31484);
#28004=AXIS2_PLACEMENT_3D('',#41527,#31485,#31486);
#28005=AXIS2_PLACEMENT_3D('',#41529,#31487,#31488);
#28006=AXIS2_PLACEMENT_3D('',#41532,#31490,#31491);
#28007=AXIS2_PLACEMENT_3D('',#41533,#31492,#31493);
#28008=AXIS2_PLACEMENT_3D('',#41536,#31494,#31495);
#28009=AXIS2_PLACEMENT_3D('',#41540,#31497,#31498);
#28010=AXIS2_PLACEMENT_3D('',#41544,#31500,#31501);
#28011=AXIS2_PLACEMENT_3D('',#41552,#31505,#31506);
#28012=AXIS2_PLACEMENT_3D('',#41555,#31508,#31509);
#28013=AXIS2_PLACEMENT_3D('',#41560,#31511,#31512);
#28014=AXIS2_PLACEMENT_3D('',#41564,#31514,#31515);
#28015=AXIS2_PLACEMENT_3D('',#41568,#31517,#31518);
#28016=AXIS2_PLACEMENT_3D('',#41571,#31520,#31521);
#28017=AXIS2_PLACEMENT_3D('',#41572,#31522,#31523);
#28018=AXIS2_PLACEMENT_3D('',#41575,#31525,#31526);
#28019=AXIS2_PLACEMENT_3D('',#41576,#31527,#31528);
#28020=AXIS2_PLACEMENT_3D('',#41579,#31530,#31531);
#28021=AXIS2_PLACEMENT_3D('',#41580,#31532,#31533);
#28022=AXIS2_PLACEMENT_3D('',#41583,#31535,#31536);
#28023=AXIS2_PLACEMENT_3D('',#41584,#31537,#31538);
#28024=AXIS2_PLACEMENT_3D('',#41589,#31540,#31541);
#28025=AXIS2_PLACEMENT_3D('',#41592,#31543,#31544);
#28026=AXIS2_PLACEMENT_3D('',#41622,#31545,#31546);
#28027=AXIS2_PLACEMENT_3D('',#41626,#31548,#31549);
#28028=AXIS2_PLACEMENT_3D('',#41631,#31552,#31553);
#28029=AXIS2_PLACEMENT_3D('',#41635,#31555,#31556);
#28030=AXIS2_PLACEMENT_3D('',#41647,#31562,#31563);
#28031=AXIS2_PLACEMENT_3D('',#41651,#31565,#31566);
#28032=AXIS2_PLACEMENT_3D('',#41655,#31568,#31569);
#28033=AXIS2_PLACEMENT_3D('',#41658,#31571,#31572);
#28034=AXIS2_PLACEMENT_3D('',#41659,#31573,#31574);
#28035=AXIS2_PLACEMENT_3D('',#41661,#31575,#31576);
#28036=AXIS2_PLACEMENT_3D('',#41663,#31578,#31579);
#28037=AXIS2_PLACEMENT_3D('',#41667,#31581,#31582);
#28038=AXIS2_PLACEMENT_3D('',#41669,#31583,#31584);
#28039=AXIS2_PLACEMENT_3D('',#41695,#31586,#31587);
#28040=AXIS2_PLACEMENT_3D('',#41698,#31589,#31590);
#28041=AXIS2_PLACEMENT_3D('',#41703,#31591,#31592);
#28042=AXIS2_PLACEMENT_3D('',#41705,#31593,#31594);
#28043=AXIS2_PLACEMENT_3D('',#41707,#31596,#31597);
#28044=AXIS2_PLACEMENT_3D('',#41711,#31599,#31600);
#28045=AXIS2_PLACEMENT_3D('',#41742,#31602,#31603);
#28046=AXIS2_PLACEMENT_3D('',#41744,#31604,#31605);
#28047=AXIS2_PLACEMENT_3D('',#41746,#31607,#31608);
#28048=AXIS2_PLACEMENT_3D('',#41750,#31610,#31611);
#28049=AXIS2_PLACEMENT_3D('',#41752,#31612,#31613);
#28050=AXIS2_PLACEMENT_3D('',#41774,#31615,#31616);
#28051=AXIS2_PLACEMENT_3D('',#41776,#31617,#31618);
#28052=AXIS2_PLACEMENT_3D('',#41778,#31620,#31621);
#28053=AXIS2_PLACEMENT_3D('',#41780,#31622,#31623);
#28054=AXIS2_PLACEMENT_3D('',#41782,#31625,#31626);
#28055=AXIS2_PLACEMENT_3D('',#41810,#31631,#31632);
#28056=AXIS2_PLACEMENT_3D('',#41812,#31633,#31634);
#28057=AXIS2_PLACEMENT_3D('',#41817,#31636,#31637);
#28058=AXIS2_PLACEMENT_3D('',#41821,#31639,#31640);
#28059=AXIS2_PLACEMENT_3D('',#41825,#31642,#31643);
#28060=AXIS2_PLACEMENT_3D('',#41828,#31645,#31646);
#28061=AXIS2_PLACEMENT_3D('',#41830,#31647,#31648);
#28062=AXIS2_PLACEMENT_3D('',#41831,#31649,#31650);
#28063=AXIS2_PLACEMENT_3D('',#41833,#31652,#31653);
#28064=AXIS2_PLACEMENT_3D('',#41835,#31655,#31656);
#28065=AXIS2_PLACEMENT_3D('',#41837,#31658,#31659);
#28066=AXIS2_PLACEMENT_3D('',#41839,#31660,#31661);
#28067=AXIS2_PLACEMENT_3D('',#41842,#31663,#31664);
#28068=AXIS2_PLACEMENT_3D('',#41843,#31665,#31666);
#28069=AXIS2_PLACEMENT_3D('',#41845,#31667,#31668);
#28070=AXIS2_PLACEMENT_3D('',#41847,#31669,#31670);
#28071=AXIS2_PLACEMENT_3D('',#41849,#31671,#31672);
#28072=AXIS2_PLACEMENT_3D('',#41851,#31673,#31674);
#28073=AXIS2_PLACEMENT_3D('',#41853,#31675,#31676);
#28074=AXIS2_PLACEMENT_3D('',#41854,#31677,#31678);
#28075=AXIS2_PLACEMENT_3D('',#41856,#31679,#31680);
#28076=AXIS2_PLACEMENT_3D('',#41858,#31682,#31683);
#28077=AXIS2_PLACEMENT_3D('',#41861,#31685,#31686);
#28078=AXIS2_PLACEMENT_3D('',#41862,#31687,#31688);
#28079=AXIS2_PLACEMENT_3D('',#41864,#31689,#31690);
#28080=AXIS2_PLACEMENT_3D('',#41866,#31692,#31693);
#28081=AXIS2_PLACEMENT_3D('',#41869,#31695,#31696);
#28082=AXIS2_PLACEMENT_3D('',#41870,#31697,#31698);
#28083=AXIS2_PLACEMENT_3D('',#41872,#31699,#31700);
#28084=AXIS2_PLACEMENT_3D('',#41874,#31702,#31703);
#28085=AXIS2_PLACEMENT_3D('',#41877,#31705,#31706);
#28086=AXIS2_PLACEMENT_3D('',#41878,#31707,#31708);
#28087=AXIS2_PLACEMENT_3D('',#41880,#31709,#31710);
#28088=AXIS2_PLACEMENT_3D('',#41882,#31712,#31713);
#28089=AXIS2_PLACEMENT_3D('',#41884,#31714,#31715);
#28090=AXIS2_PLACEMENT_3D('',#41886,#31717,#31718);
#28091=AXIS2_PLACEMENT_3D('',#41891,#31720,#31721);
#28092=AXIS2_PLACEMENT_3D('',#41895,#31723,#31724);
#28093=AXIS2_PLACEMENT_3D('',#41899,#31726,#31727);
#28094=AXIS2_PLACEMENT_3D('',#41902,#31729,#31730);
#28095=AXIS2_PLACEMENT_3D('',#41904,#31731,#31732);
#28096=AXIS2_PLACEMENT_3D('',#41905,#31733,#31734);
#28097=AXIS2_PLACEMENT_3D('',#41907,#31736,#31737);
#28098=AXIS2_PLACEMENT_3D('',#41909,#31738,#31739);
#28099=AXIS2_PLACEMENT_3D('',#41911,#31740,#31741);
#28100=AXIS2_PLACEMENT_3D('',#41912,#31742,#31743);
#28101=AXIS2_PLACEMENT_3D('',#41913,#31744,#31745);
#28102=AXIS2_PLACEMENT_3D('',#41916,#31747,#31748);
#28103=AXIS2_PLACEMENT_3D('',#41917,#31749,#31750);
#28104=AXIS2_PLACEMENT_3D('',#41919,#31751,#31752);
#28105=AXIS2_PLACEMENT_3D('',#41921,#31753,#31754);
#28106=AXIS2_PLACEMENT_3D('',#41923,#31755,#31756);
#28107=AXIS2_PLACEMENT_3D('',#41925,#31757,#31758);
#28108=AXIS2_PLACEMENT_3D('',#41927,#31759,#31760);
#28109=AXIS2_PLACEMENT_3D('',#41928,#31761,#31762);
#28110=AXIS2_PLACEMENT_3D('',#41930,#31763,#31764);
#28111=AXIS2_PLACEMENT_3D('',#41931,#31765,#31766);
#28112=AXIS2_PLACEMENT_3D('',#41932,#31767,#31768);
#28113=AXIS2_PLACEMENT_3D('',#41934,#31769,#31770);
#28114=AXIS2_PLACEMENT_3D('',#41936,#31771,#31772);
#28115=AXIS2_PLACEMENT_3D('',#41938,#31773,#31774);
#28116=AXIS2_PLACEMENT_3D('',#41940,#31775,#31776);
#28117=AXIS2_PLACEMENT_3D('',#41942,#31777,#31778);
#28118=AXIS2_PLACEMENT_3D('',#41943,#31779,#31780);
#28119=AXIS2_PLACEMENT_3D('',#41945,#31781,#31782);
#28120=AXIS2_PLACEMENT_3D('',#41947,#31783,#31784);
#28121=AXIS2_PLACEMENT_3D('',#41948,#31785,#31786);
#28122=AXIS2_PLACEMENT_3D('',#41949,#31787,#31788);
#28123=AXIS2_PLACEMENT_3D('',#41952,#31790,#31791);
#28124=AXIS2_PLACEMENT_3D('',#41953,#31792,#31793);
#28125=AXIS2_PLACEMENT_3D('',#41954,#31794,#31795);
#28126=AXIS2_PLACEMENT_3D('',#41956,#31797,#31798);
#28127=AXIS2_PLACEMENT_3D('',#41958,#31799,#31800);
#28128=AXIS2_PLACEMENT_3D('',#41959,#31801,#31802);
#28129=AXIS2_PLACEMENT_3D('',#41960,#31803,#31804);
#28130=AXIS2_PLACEMENT_3D('',#41964,#31806,#31807);
#28131=AXIS2_PLACEMENT_3D('',#41998,#31808,#31809);
#28132=AXIS2_PLACEMENT_3D('',#42015,#31810,#31811);
#28133=AXIS2_PLACEMENT_3D('',#42036,#31812,#31813);
#28134=AXIS2_PLACEMENT_3D('',#42075,#31814,#31815);
#28135=AXIS2_PLACEMENT_3D('',#42076,#31816,#31817);
#28136=AXIS2_PLACEMENT_3D('',#42083,#31818,#31819);
#28137=AXIS2_PLACEMENT_3D('',#42088,#31820,#31821);
#28138=AXIS2_PLACEMENT_3D('',#42090,#31823,#31824);
#28139=AXIS2_PLACEMENT_3D('',#42097,#31825,#31826);
#28140=AXIS2_PLACEMENT_3D('',#42102,#31827,#31828);
#28141=AXIS2_PLACEMENT_3D('',#42104,#31830,#31831);
#28142=AXIS2_PLACEMENT_3D('',#42105,#31832,#31833);
#28143=AXIS2_PLACEMENT_3D('',#42106,#31834,#31835);
#28144=AXIS2_PLACEMENT_3D('',#42107,#31836,#31837);
#28145=AXIS2_PLACEMENT_3D('',#42109,#31838,#31839);
#28146=AXIS2_PLACEMENT_3D('',#42111,#31840,#31841);
#28147=AXIS2_PLACEMENT_3D('',#42123,#31843,#31844);
#28148=AXIS2_PLACEMENT_3D('',#42124,#31845,#31846);
#28149=AXIS2_PLACEMENT_3D('',#42125,#31847,#31848);
#28150=AXIS2_PLACEMENT_3D('',#42127,#31849,#31850);
#28151=AXIS2_PLACEMENT_3D('',#42139,#31852,#31853);
#28152=AXIS2_PLACEMENT_3D('',#42140,#31854,#31855);
#28153=AXIS2_PLACEMENT_3D('',#42141,#31856,#31857);
#28154=AXIS2_PLACEMENT_3D('',#42143,#31858,#31859);
#28155=AXIS2_PLACEMENT_3D('',#42155,#31861,#31862);
#28156=AXIS2_PLACEMENT_3D('',#42156,#31863,#31864);
#28157=AXIS2_PLACEMENT_3D('',#42157,#31865,#31866);
#28158=AXIS2_PLACEMENT_3D('',#42159,#31867,#31868);
#28159=AXIS2_PLACEMENT_3D('',#42170,#31870,#31871);
#28160=AXIS2_PLACEMENT_3D('',#42171,#31872,#31873);
#28161=AXIS2_PLACEMENT_3D('',#42174,#31876,#31877);
#28162=AXIS2_PLACEMENT_3D('',#42176,#31879,#31880);
#28163=AXIS2_PLACEMENT_3D('',#42178,#31882,#31883);
#28164=AXIS2_PLACEMENT_3D('',#42180,#31885,#31886);
#28165=AXIS2_PLACEMENT_3D('',#42182,#31887,#31888);
#28166=AXIS2_PLACEMENT_3D('',#42183,#31889,#31890);
#28167=AXIS2_PLACEMENT_3D('',#42184,#31891,#31892);
#28168=AXIS2_PLACEMENT_3D('',#42187,#31895,#31896);
#28169=AXIS2_PLACEMENT_3D('',#42189,#31897,#31898);
#28170=AXIS2_PLACEMENT_3D('',#42191,#31899,#31900);
#28171=AXIS2_PLACEMENT_3D('',#42192,#31901,#31902);
#28172=AXIS2_PLACEMENT_3D('',#42194,#31903,#31904);
#28173=AXIS2_PLACEMENT_3D('',#42196,#31905,#31906);
#28174=AXIS2_PLACEMENT_3D('',#42197,#31907,#31908);
#28175=AXIS2_PLACEMENT_3D('',#42198,#31909,#31910);
#28176=AXIS2_PLACEMENT_3D('',#42202,#31912,#31913);
#28177=AXIS2_PLACEMENT_3D('',#42204,#31915,#31916);
#28178=AXIS2_PLACEMENT_3D('',#42208,#31918,#31919);
#28179=AXIS2_PLACEMENT_3D('',#42210,#31921,#31922);
#28180=AXIS2_PLACEMENT_3D('',#42212,#31924,#31925);
#28181=AXIS2_PLACEMENT_3D('',#42215,#31927,#31928);
#28182=AXIS2_PLACEMENT_3D('',#42216,#31929,#31930);
#28183=AXIS2_PLACEMENT_3D('',#42218,#31931,#31932);
#28184=AXIS2_PLACEMENT_3D('',#42220,#31934,#31935);
#28185=AXIS2_PLACEMENT_3D('',#42222,#31936,#31937);
#28186=AXIS2_PLACEMENT_3D('',#42224,#31938,#31939);
#28187=AXIS2_PLACEMENT_3D('',#42225,#31940,#31941);
#28188=AXIS2_PLACEMENT_3D('',#42226,#31942,#31943);
#28189=AXIS2_PLACEMENT_3D('',#42228,#31944,#31945);
#28190=AXIS2_PLACEMENT_3D('',#42230,#31947,#31948);
#28191=AXIS2_PLACEMENT_3D('',#42232,#31949,#31950);
#28192=AXIS2_PLACEMENT_3D('',#42233,#31951,#31952);
#28193=AXIS2_PLACEMENT_3D('',#42234,#31953,#31954);
#28194=AXIS2_PLACEMENT_3D('',#42235,#31955,#31956);
#28195=AXIS2_PLACEMENT_3D('',#42238,#31957,#31958);
#28196=AXIS2_PLACEMENT_3D('',#42242,#31960,#31961);
#28197=AXIS2_PLACEMENT_3D('',#42244,#31963,#31964);
#28198=AXIS2_PLACEMENT_3D('',#42247,#31965,#31966);
#28199=AXIS2_PLACEMENT_3D('',#42248,#31967,#31968);
#28200=AXIS2_PLACEMENT_3D('',#42249,#31969,#31970);
#28201=AXIS2_PLACEMENT_3D('',#42250,#31971,#31972);
#28202=AXIS2_PLACEMENT_3D('',#42253,#31973,#31974);
#28203=AXIS2_PLACEMENT_3D('',#42256,#31977,#31978);
#28204=AXIS2_PLACEMENT_3D('',#42259,#31979,#31980);
#28205=AXIS2_PLACEMENT_3D('',#42260,#31981,#31982);
#28206=AXIS2_PLACEMENT_3D('',#42261,#31983,#31984);
#28207=AXIS2_PLACEMENT_3D('',#42262,#31985,#31986);
#28208=AXIS2_PLACEMENT_3D('',#42265,#31987,#31988);
#28209=AXIS2_PLACEMENT_3D('',#42268,#31991,#31992);
#28210=AXIS2_PLACEMENT_3D('',#42271,#31993,#31994);
#28211=AXIS2_PLACEMENT_3D('',#42272,#31995,#31996);
#28212=AXIS2_PLACEMENT_3D('',#42273,#31997,#31998);
#28213=AXIS2_PLACEMENT_3D('',#42274,#31999,#32000);
#28214=AXIS2_PLACEMENT_3D('',#42277,#32001,#32002);
#28215=AXIS2_PLACEMENT_3D('',#42280,#32005,#32006);
#28216=AXIS2_PLACEMENT_3D('',#42281,#32007,#32008);
#28217=AXIS2_PLACEMENT_3D('',#42282,#32009,#32010);
#28218=AXIS2_PLACEMENT_3D('',#42283,#32011,#32012);
#28219=AXIS2_PLACEMENT_3D('',#42287,#32014,#32015);
#28220=AXIS2_PLACEMENT_3D('',#42289,#32017,#32018);
#28221=AXIS2_PLACEMENT_3D('',#42293,#32021,#32022);
#28222=AXIS2_PLACEMENT_3D('',#42296,#32024,#32025);
#28223=AXIS2_PLACEMENT_3D('',#42297,#32026,#32027);
#28224=AXIS2_PLACEMENT_3D('',#42301,#32030,#32031);
#28225=AXIS2_PLACEMENT_3D('',#42307,#32035,#32036);
#28226=AXIS2_PLACEMENT_3D('',#42309,#32037,#32038);
#28227=AXIS2_PLACEMENT_3D('',#42311,#32039,#32040);
#28228=AXIS2_PLACEMENT_3D('',#42313,#32042,#32043);
#28229=AXIS2_PLACEMENT_3D('',#42316,#32044,#32045);
#28230=AXIS2_PLACEMENT_3D('',#42317,#32046,#32047);
#28231=AXIS2_PLACEMENT_3D('',#42318,#32048,#32049);
#28232=AXIS2_PLACEMENT_3D('',#42319,#32050,#32051);
#28233=AXIS2_PLACEMENT_3D('',#42322,#32052,#32053);
#28234=AXIS2_PLACEMENT_3D('',#42325,#32056,#32057);
#28235=AXIS2_PLACEMENT_3D('',#42328,#32058,#32059);
#28236=AXIS2_PLACEMENT_3D('',#42329,#32060,#32061);
#28237=AXIS2_PLACEMENT_3D('',#42330,#32062,#32063);
#28238=AXIS2_PLACEMENT_3D('',#42331,#32064,#32065);
#28239=AXIS2_PLACEMENT_3D('',#42333,#32066,#32067);
#28240=AXIS2_PLACEMENT_3D('',#42336,#32070,#32071);
#28241=AXIS2_PLACEMENT_3D('',#42338,#32072,#32073);
#28242=AXIS2_PLACEMENT_3D('',#42339,#32074,#32075);
#28243=AXIS2_PLACEMENT_3D('',#42340,#32076,#32077);
#28244=AXIS2_PLACEMENT_3D('',#42342,#32078,#32079);
#28245=AXIS2_PLACEMENT_3D('',#42344,#32081,#32082);
#28246=AXIS2_PLACEMENT_3D('',#42345,#32083,#32084);
#28247=AXIS2_PLACEMENT_3D('',#42346,#32085,#32086);
#28248=AXIS2_PLACEMENT_3D('',#42349,#32089,#32090);
#28249=AXIS2_PLACEMENT_3D('',#42351,#32092,#32093);
#28250=AXIS2_PLACEMENT_3D('',#42352,#32094,#32095);
#28251=AXIS2_PLACEMENT_3D('',#42355,#32098,#32099);
#28252=AXIS2_PLACEMENT_3D('',#42357,#32100,#32101);
#28253=AXIS2_PLACEMENT_3D('',#42359,#32102,#32103);
#28254=AXIS2_PLACEMENT_3D('',#42361,#32105,#32106);
#28255=AXIS2_PLACEMENT_3D('',#42364,#32107,#32108);
#28256=AXIS2_PLACEMENT_3D('',#42365,#32109,#32110);
#28257=AXIS2_PLACEMENT_3D('',#42366,#32111,#32112);
#28258=AXIS2_PLACEMENT_3D('',#42367,#32113,#32114);
#28259=AXIS2_PLACEMENT_3D('',#42370,#32115,#32116);
#28260=AXIS2_PLACEMENT_3D('',#42373,#32119,#32120);
#28261=AXIS2_PLACEMENT_3D('',#42375,#32121,#32122);
#28262=AXIS2_PLACEMENT_3D('',#42376,#32123,#32124);
#28263=AXIS2_PLACEMENT_3D('',#42377,#32125,#32126);
#28264=AXIS2_PLACEMENT_3D('',#42378,#32127,#32128);
#28265=AXIS2_PLACEMENT_3D('',#42380,#32129,#32130);
#28266=AXIS2_PLACEMENT_3D('',#42382,#32132,#32133);
#28267=AXIS2_PLACEMENT_3D('',#42385,#32134,#32135);
#28268=AXIS2_PLACEMENT_3D('',#42386,#32136,#32137);
#28269=AXIS2_PLACEMENT_3D('',#42387,#32138,#32139);
#28270=AXIS2_PLACEMENT_3D('',#42388,#32140,#32141);
#28271=AXIS2_PLACEMENT_3D('',#42391,#32142,#32143);
#28272=AXIS2_PLACEMENT_3D('',#42394,#32146,#32147);
#28273=AXIS2_PLACEMENT_3D('',#42395,#32148,#32149);
#28274=AXIS2_PLACEMENT_3D('',#42396,#32150,#32151);
#28275=AXIS2_PLACEMENT_3D('',#42397,#32152,#32153);
#28276=AXIS2_PLACEMENT_3D('',#42399,#32155,#32156);
#28277=AXIS2_PLACEMENT_3D('',#42402,#32158,#32159);
#28278=AXIS2_PLACEMENT_3D('',#42406,#32161,#32162);
#28279=AXIS2_PLACEMENT_3D('',#42410,#32164,#32165);
#28280=AXIS2_PLACEMENT_3D('',#42413,#32167,#32168);
#28281=AXIS2_PLACEMENT_3D('',#42414,#32169,#32170);
#28282=AXIS2_PLACEMENT_3D('',#42415,#32171,#32172);
#28283=AXIS2_PLACEMENT_3D('',#42417,#32173,#32174);
#28284=AXIS2_PLACEMENT_3D('',#42418,#32175,#32176);
#28285=AXIS2_PLACEMENT_3D('',#42420,#32177,#32178);
#28286=AXIS2_PLACEMENT_3D('',#42423,#32180,#32181);
#28287=AXIS2_PLACEMENT_3D('',#42424,#32182,#32183);
#28288=AXIS2_PLACEMENT_3D('',#42426,#32184,#32185);
#28289=AXIS2_PLACEMENT_3D('',#42427,#32186,#32187);
#28290=AXIS2_PLACEMENT_3D('',#42428,#32188,#32189);
#28291=AXIS2_PLACEMENT_3D('',#42430,#32190,#32191);
#28292=AXIS2_PLACEMENT_3D('',#42432,#32193,#32194);
#28293=AXIS2_PLACEMENT_3D('',#42434,#32195,#32196);
#28294=AXIS2_PLACEMENT_3D('',#42435,#32197,#32198);
#28295=AXIS2_PLACEMENT_3D('',#42436,#32199,#32200);
#28296=AXIS2_PLACEMENT_3D('',#42438,#32201,#32202);
#28297=AXIS2_PLACEMENT_3D('',#42440,#32204,#32205);
#28298=AXIS2_PLACEMENT_3D('',#42442,#32206,#32207);
#28299=AXIS2_PLACEMENT_3D('',#42443,#32208,#32209);
#28300=AXIS2_PLACEMENT_3D('',#42444,#32210,#32211);
#28301=AXIS2_PLACEMENT_3D('',#42446,#32212,#32213);
#28302=AXIS2_PLACEMENT_3D('',#42448,#32215,#32216);
#28303=AXIS2_PLACEMENT_3D('',#42449,#32217,#32218);
#28304=AXIS2_PLACEMENT_3D('',#42450,#32219,#32220);
#28305=AXIS2_PLACEMENT_3D('',#42454,#32222,#32223);
#28306=AXIS2_PLACEMENT_3D('',#42456,#32225,#32226);
#28307=AXIS2_PLACEMENT_3D('',#42460,#32229,#32230);
#28308=AXIS2_PLACEMENT_3D('',#42463,#32232,#32233);
#28309=AXIS2_PLACEMENT_3D('',#42464,#32234,#32235);
#28310=AXIS2_PLACEMENT_3D('',#42468,#32238,#32239);
#28311=AXIS2_PLACEMENT_3D('',#42469,#32240,#32241);
#28312=AXIS2_PLACEMENT_3D('',#42470,#32242,#32243);
#28313=AXIS2_PLACEMENT_3D('',#42471,#32244,#32245);
#28314=AXIS2_PLACEMENT_3D('',#42473,#32246,#32247);
#28315=AXIS2_PLACEMENT_3D('',#42474,#32248,#32249);
#28316=AXIS2_PLACEMENT_3D('',#42475,#32250,#32251);
#28317=AXIS2_PLACEMENT_3D('',#42477,#32252,#32253);
#28318=AXIS2_PLACEMENT_3D('',#42479,#32255,#32256);
#28319=AXIS2_PLACEMENT_3D('',#42481,#32257,#32258);
#28320=AXIS2_PLACEMENT_3D('',#42482,#32259,#32260);
#28321=AXIS2_PLACEMENT_3D('',#42483,#32261,#32262);
#28322=AXIS2_PLACEMENT_3D('',#42484,#32263,#32264);
#28323=AXIS2_PLACEMENT_3D('',#42486,#32266,#32267);
#28324=AXIS2_PLACEMENT_3D('',#42487,#32268,#32269);
#28325=AXIS2_PLACEMENT_3D('',#42488,#32270,#32271);
#28326=AXIS2_PLACEMENT_3D('',#42489,#32272,#32273);
#28327=AXIS2_PLACEMENT_3D('',#42490,#32274,#32275);
#28328=AXIS2_PLACEMENT_3D('',#42491,#32276,#32277);
#28329=AXIS2_PLACEMENT_3D('',#42494,#32280,#32281);
#28330=AXIS2_PLACEMENT_3D('',#42496,#32283,#32284);
#28331=AXIS2_PLACEMENT_3D('',#42497,#32285,#32286);
#28332=AXIS2_PLACEMENT_3D('',#42498,#32287,#32288);
#28333=AXIS2_PLACEMENT_3D('',#42499,#32289,#32290);
#28334=AXIS2_PLACEMENT_3D('',#42500,#32291,#32292);
#28335=AXIS2_PLACEMENT_3D('',#42501,#32293,#32294);
#28336=AXIS2_PLACEMENT_3D('',#42503,#32296,#32297);
#28337=AXIS2_PLACEMENT_3D('',#42505,#32299,#32300);
#28338=AXIS2_PLACEMENT_3D('',#42507,#32302,#32303);
#28339=AXIS2_PLACEMENT_3D('',#42509,#32305,#32306);
#28340=AXIS2_PLACEMENT_3D('',#42510,#32307,#32308);
#28341=AXIS2_PLACEMENT_3D('',#42511,#32309,#32310);
#28342=AXIS2_PLACEMENT_3D('',#42513,#32311,#32312);
#28343=AXIS2_PLACEMENT_3D('',#42515,#32313,#32314);
#28344=AXIS2_PLACEMENT_3D('',#42516,#32315,#32316);
#28345=AXIS2_PLACEMENT_3D('',#42518,#32318,#32319);
#28346=AXIS2_PLACEMENT_3D('',#42520,#32320,#32321);
#28347=AXIS2_PLACEMENT_3D('',#42522,#32322,#32323);
#28348=AXIS2_PLACEMENT_3D('',#42523,#32324,#32325);
#28349=AXIS2_PLACEMENT_3D('',#42525,#32327,#32328);
#28350=AXIS2_PLACEMENT_3D('',#42527,#32330,#32331);
#28351=AXIS2_PLACEMENT_3D('',#42529,#32333,#32334);
#28352=AXIS2_PLACEMENT_3D('',#42530,#32335,#32336);
#28353=AXIS2_PLACEMENT_3D('',#42532,#32338,#32339);
#28354=AXIS2_PLACEMENT_3D('',#42533,#32340,#32341);
#28355=AXIS2_PLACEMENT_3D('',#42535,#32343,#32344);
#28356=AXIS2_PLACEMENT_3D('',#42537,#32346,#32347);
#28357=AXIS2_PLACEMENT_3D('',#42539,#32349,#32350);
#28358=AXIS2_PLACEMENT_3D('',#42540,#32351,#32352);
#28359=AXIS2_PLACEMENT_3D('',#42543,#32355,#32356);
#28360=AXIS2_PLACEMENT_3D('',#42545,#32358,#32359);
#28361=AXIS2_PLACEMENT_3D('',#42547,#32361,#32362);
#28362=AXIS2_PLACEMENT_3D('',#42549,#32364,#32365);
#28363=AXIS2_PLACEMENT_3D('',#42551,#32367,#32368);
#28364=AXIS2_PLACEMENT_3D('',#42553,#32370,#32371);
#28365=AXIS2_PLACEMENT_3D('',#42555,#32373,#32374);
#28366=AXIS2_PLACEMENT_3D('',#42556,#32375,#32376);
#28367=AXIS2_PLACEMENT_3D('',#42559,#32379,#32380);
#28368=AXIS2_PLACEMENT_3D('',#42560,#32381,#32382);
#28369=AXIS2_PLACEMENT_3D('',#42561,#32383,#32384);
#28370=AXIS2_PLACEMENT_3D('',#42563,#32386,#32387);
#31448=DIRECTION('axis',(0.,0.,1.));
#31449=DIRECTION('refdir',(1.,0.,0.));
#31450=DIRECTION('center_axis',(0.,1.,0.));
#31451=DIRECTION('ref_axis',(0.,0.,1.));
#31452=DIRECTION('center_axis',(0.,1.,0.));
#31453=DIRECTION('ref_axis',(0.,0.,1.));
#31454=DIRECTION('',(8.65956056235486E-17,-0.707106781186554,0.707106781186541));
#31455=DIRECTION('center_axis',(0.,-1.,0.));
#31456=DIRECTION('ref_axis',(0.,0.,1.));
#31457=DIRECTION('center_axis',(0.,1.,0.));
#31458=DIRECTION('ref_axis',(0.,0.,1.));
#31459=DIRECTION('center_axis',(0.,1.,0.));
#31460=DIRECTION('ref_axis',(0.,0.,1.));
#31461=DIRECTION('',(0.,1.,0.));
#31462=DIRECTION('center_axis',(0.,1.,0.));
#31463=DIRECTION('ref_axis',(1.,0.,0.));
#31464=DIRECTION('center_axis',(0.,1.,0.));
#31465=DIRECTION('ref_axis',(1.,0.,-2.96059473233374E-15));
#31466=DIRECTION('',(1.,0.,0.));
#31467=DIRECTION('center_axis',(0.,1.,0.));
#31468=DIRECTION('ref_axis',(-2.96059473233374E-15,0.,-1.));
#31469=DIRECTION('',(0.,0.,-1.));
#31470=DIRECTION('center_axis',(0.,1.,0.));
#31471=DIRECTION('ref_axis',(-1.,0.,2.96059473233374E-15));
#31472=DIRECTION('',(-1.,0.,0.));
#31473=DIRECTION('center_axis',(0.,1.,0.));
#31474=DIRECTION('ref_axis',(2.96059473233374E-15,0.,1.));
#31475=DIRECTION('',(0.,0.,1.));
#31476=DIRECTION('center_axis',(0.,-1.,0.));
#31477=DIRECTION('ref_axis',(0.,0.,1.));
#31478=DIRECTION('',(-8.65956056235486E-17,-0.707106781186554,-0.707106781186541));
#31479=DIRECTION('center_axis',(0.,-1.,0.));
#31480=DIRECTION('ref_axis',(0.,0.,1.));
#31481=DIRECTION('center_axis',(0.,1.,0.));
#31482=DIRECTION('ref_axis',(0.,0.,1.));
#31483=DIRECTION('center_axis',(0.,1.,0.));
#31484=DIRECTION('ref_axis',(1.,0.,0.));
#31485=DIRECTION('center_axis',(0.,0.,1.));
#31486=DIRECTION('ref_axis',(1.,0.,0.));
#31487=DIRECTION('center_axis',(0.,0.,1.));
#31488=DIRECTION('ref_axis',(1.,0.,0.));
#31489=DIRECTION('',(0.707106781186541,8.65956056235486E-17,-0.707106781186554));
#31490=DIRECTION('center_axis',(0.,0.,-1.));
#31491=DIRECTION('ref_axis',(1.,0.,0.));
#31492=DIRECTION('center_axis',(0.,0.,1.));
#31493=DIRECTION('ref_axis',(1.,0.,0.));
#31494=DIRECTION('center_axis',(0.,0.,1.));
#31495=DIRECTION('ref_axis',(-1.,0.,0.));
#31496=DIRECTION('',(1.,0.,0.));
#31497=DIRECTION('center_axis',(0.,0.,1.));
#31498=DIRECTION('ref_axis',(0.,-1.,0.));
#31499=DIRECTION('',(0.,1.,0.));
#31500=DIRECTION('center_axis',(0.,0.,1.));
#31501=DIRECTION('ref_axis',(1.,0.,0.));
#31502=DIRECTION('',(-1.,0.,0.));
#31503=DIRECTION('',(0.,1.,0.));
#31504=DIRECTION('',(-1.,0.,0.));
#31505=DIRECTION('center_axis',(0.,0.,1.));
#31506=DIRECTION('ref_axis',(0.,1.,0.));
#31507=DIRECTION('',(0.,-1.,0.));
#31508=DIRECTION('center_axis',(0.,0.,1.));
#31509=DIRECTION('ref_axis',(1.,0.,0.));
#31510=DIRECTION('',(1.,0.,0.));
#31511=DIRECTION('center_axis',(0.,0.,1.));
#31512=DIRECTION('ref_axis',(-1.,0.,0.));
#31513=DIRECTION('',(0.,-1.,0.));
#31514=DIRECTION('center_axis',(0.,0.,1.));
#31515=DIRECTION('ref_axis',(4.44089209850064E-15,1.,0.));
#31516=DIRECTION('',(-1.,0.,0.));
#31517=DIRECTION('center_axis',(0.,0.,1.));
#31518=DIRECTION('ref_axis',(1.,0.,0.));
#31519=DIRECTION('',(0.,1.,0.));
#31520=DIRECTION('center_axis',(0.,0.,1.));
#31521=DIRECTION('ref_axis',(-4.44089209850064E-15,-1.,0.));
#31522=DIRECTION('center_axis',(0.,0.,-1.));
#31523=DIRECTION('ref_axis',(1.,0.,0.));
#31524=DIRECTION('',(0.,0.,-1.));
#31525=DIRECTION('center_axis',(0.,0.,1.));
#31526=DIRECTION('ref_axis',(1.,0.,0.));
#31527=DIRECTION('center_axis',(0.,0.,1.));
#31528=DIRECTION('ref_axis',(1.,0.,0.));
#31529=DIRECTION('',(0.707106781186541,8.65956056235486E-17,-0.707106781186554));
#31530=DIRECTION('center_axis',(0.,0.,-1.));
#31531=DIRECTION('ref_axis',(1.,0.,0.));
#31532=DIRECTION('center_axis',(0.,0.,-1.));
#31533=DIRECTION('ref_axis',(1.,0.,0.));
#31534=DIRECTION('',(0.,0.,-1.));
#31535=DIRECTION('center_axis',(0.,0.,1.));
#31536=DIRECTION('ref_axis',(1.,0.,0.));
#31537=DIRECTION('center_axis',(1.,0.,0.));
#31538=DIRECTION('ref_axis',(0.,0.,-1.));
#31539=DIRECTION('',(-0.707106781186546,-0.127511058902472,-0.695514866740871));
#31540=DIRECTION('center_axis',(-1.,0.,0.));
#31541=DIRECTION('ref_axis',(0.,0.,-1.));
#31542=DIRECTION('',(0.707106781186546,-0.127511058902472,0.695514866740871));
#31543=DIRECTION('center_axis',(1.,0.,0.));
#31544=DIRECTION('ref_axis',(0.,0.,-1.));
#31545=DIRECTION('center_axis',(-1.,0.,0.));
#31546=DIRECTION('ref_axis',(0.,0.,1.));
#31547=DIRECTION('',(0.,1.,0.));
#31548=DIRECTION('center_axis',(1.,0.,0.));
#31549=DIRECTION('ref_axis',(0.,0.,-1.));
#31550=DIRECTION('',(0.,1.,0.));
#31551=DIRECTION('',(0.,1.,0.));
#31552=DIRECTION('center_axis',(1.,0.,0.));
#31553=DIRECTION('ref_axis',(0.,0.,-1.));
#31554=DIRECTION('',(0.,1.,0.));
#31555=DIRECTION('center_axis',(1.,0.,0.));
#31556=DIRECTION('ref_axis',(0.,0.,-1.));
#31557=DIRECTION('',(0.,1.,0.));
#31558=DIRECTION('',(0.,0.,1.));
#31559=DIRECTION('',(0.,0.,1.));
#31560=DIRECTION('',(0.,1.,0.));
#31561=DIRECTION('',(0.,0.,1.));
#31562=DIRECTION('center_axis',(1.,0.,0.));
#31563=DIRECTION('ref_axis',(0.,0.707106781186548,-0.707106781186547));
#31564=DIRECTION('',(0.,1.,0.));
#31565=DIRECTION('center_axis',(1.,0.,0.));
#31566=DIRECTION('ref_axis',(0.,-0.707106781186547,-0.707106781186548));
#31567=DIRECTION('',(0.,0.,-1.));
#31568=DIRECTION('center_axis',(1.,0.,0.));
#31569=DIRECTION('ref_axis',(0.,-0.707106781186548,0.707106781186548));
#31570=DIRECTION('',(0.,-1.,0.));
#31571=DIRECTION('center_axis',(1.,0.,0.));
#31572=DIRECTION('ref_axis',(0.,0.707106781186548,0.707106781186547));
#31573=DIRECTION('center_axis',(1.,0.,0.));
#31574=DIRECTION('ref_axis',(0.,0.,-1.));
#31575=DIRECTION('center_axis',(1.,0.,0.));
#31576=DIRECTION('ref_axis',(0.,0.,-1.));
#31577=DIRECTION('',(1.,0.,0.));
#31578=DIRECTION('center_axis',(1.,0.,0.));
#31579=DIRECTION('ref_axis',(0.,-1.22464679914735E-16,1.));
#31580=DIRECTION('',(-0.707106781186544,0.127511058902497,0.695514866740869));
#31581=DIRECTION('center_axis',(-1.,0.,0.));
#31582=DIRECTION('ref_axis',(0.,0.,-1.));
#31583=DIRECTION('center_axis',(-1.,0.,0.));
#31584=DIRECTION('ref_axis',(0.,0.,-1.));
#31585=DIRECTION('',(0.707106781186544,0.127511058902497,-0.695514866740869));
#31586=DIRECTION('center_axis',(0.,1.,0.));
#31587=DIRECTION('ref_axis',(-2.96059473233374E-15,0.,-1.));
#31588=DIRECTION('',(0.,1.,0.));
#31589=DIRECTION('center_axis',(0.,1.,0.));
#31590=DIRECTION('ref_axis',(-2.96059473233374E-15,0.,-1.));
#31591=DIRECTION('center_axis',(1.,0.,0.));
#31592=DIRECTION('ref_axis',(0.,0.,-1.));
#31593=DIRECTION('center_axis',(1.,0.,0.));
#31594=DIRECTION('ref_axis',(0.,0.,-1.));
#31595=DIRECTION('',(1.,0.,0.));
#31596=DIRECTION('center_axis',(1.,0.,0.));
#31597=DIRECTION('ref_axis',(0.,0.,-1.));
#31598=DIRECTION('',(-0.707106781186544,-0.127511058902497,-0.695514866740869));
#31599=DIRECTION('center_axis',(-1.,0.,0.));
#31600=DIRECTION('ref_axis',(0.,0.,-1.));
#31601=DIRECTION('',(0.707106781186544,-0.127511058902497,0.695514866740869));
#31602=DIRECTION('center_axis',(1.,0.,0.));
#31603=DIRECTION('ref_axis',(0.,0.,-1.));
#31604=DIRECTION('center_axis',(1.,0.,0.));
#31605=DIRECTION('ref_axis',(0.,0.,-1.));
#31606=DIRECTION('',(1.,0.,0.));
#31607=DIRECTION('center_axis',(1.,0.,0.));
#31608=DIRECTION('ref_axis',(0.,-1.22464679914735E-16,1.));
#31609=DIRECTION('',(-0.707106781186546,0.127511058902472,0.695514866740871));
#31610=DIRECTION('center_axis',(-1.,0.,0.));
#31611=DIRECTION('ref_axis',(0.,0.,-1.));
#31612=DIRECTION('center_axis',(-1.,0.,0.));
#31613=DIRECTION('ref_axis',(0.,0.,-1.));
#31614=DIRECTION('',(0.707106781186546,0.127511058902472,-0.695514866740871));
#31615=DIRECTION('center_axis',(1.,0.,0.));
#31616=DIRECTION('ref_axis',(0.,0.,-1.));
#31617=DIRECTION('center_axis',(1.,0.,0.));
#31618=DIRECTION('ref_axis',(0.,0.,-1.));
#31619=DIRECTION('',(1.,0.,0.));
#31620=DIRECTION('center_axis',(-1.,0.,0.));
#31621=DIRECTION('ref_axis',(0.,0.,-1.));
#31622=DIRECTION('center_axis',(-1.,0.,0.));
#31623=DIRECTION('ref_axis',(0.,0.,-1.));
#31624=DIRECTION('',(0.707106781186548,-8.65956056235493E-17,-0.707106781186548));
#31625=DIRECTION('center_axis',(-1.,0.,0.));
#31626=DIRECTION('ref_axis',(0.,0.,1.));
#31627=DIRECTION('',(0.,0.,-1.));
#31628=DIRECTION('',(0.,1.,0.));
#31629=DIRECTION('',(0.,0.,-1.));
#31630=DIRECTION('',(0.,1.,0.));
#31631=DIRECTION('center_axis',(-1.,0.,0.));
#31632=DIRECTION('ref_axis',(0.,0.,-1.));
#31633=DIRECTION('center_axis',(-1.,0.,0.));
#31634=DIRECTION('ref_axis',(0.,0.,-1.));
#31635=DIRECTION('',(0.,0.,-1.));
#31636=DIRECTION('center_axis',(-1.,0.,0.));
#31637=DIRECTION('ref_axis',(0.,0.707106781186548,0.707106781186547));
#31638=DIRECTION('',(0.,1.,0.));
#31639=DIRECTION('center_axis',(-1.,0.,0.));
#31640=DIRECTION('ref_axis',(0.,-0.707106781186548,0.707106781186548));
#31641=DIRECTION('',(0.,0.,1.));
#31642=DIRECTION('center_axis',(-1.,0.,0.));
#31643=DIRECTION('ref_axis',(0.,-0.707106781186547,-0.707106781186548));
#31644=DIRECTION('',(0.,-1.,0.));
#31645=DIRECTION('center_axis',(-1.,0.,0.));
#31646=DIRECTION('ref_axis',(0.,0.707106781186548,-0.707106781186547));
#31647=DIRECTION('center_axis',(-1.,0.,0.));
#31648=DIRECTION('ref_axis',(0.,0.,-1.));
#31649=DIRECTION('center_axis',(-1.,0.,0.));
#31650=DIRECTION('ref_axis',(0.,0.,-1.));
#31651=DIRECTION('',(0.707106781186548,-8.65956056235493E-17,-0.707106781186548));
#31652=DIRECTION('center_axis',(-1.,0.,0.));
#31653=DIRECTION('ref_axis',(0.,0.,-1.));
#31654=DIRECTION('',(0.707106781186548,-8.65956056235493E-17,-0.707106781186548));
#31655=DIRECTION('center_axis',(-1.,0.,0.));
#31656=DIRECTION('ref_axis',(0.,0.,-1.));
#31657=DIRECTION('',(0.707106781186548,-8.65956056235493E-17,-0.707106781186548));
#31658=DIRECTION('center_axis',(0.,1.,0.));
#31659=DIRECTION('ref_axis',(1.,0.,0.));
#31660=DIRECTION('center_axis',(0.,1.,0.));
#31661=DIRECTION('ref_axis',(1.,0.,0.));
#31662=DIRECTION('',(0.707106781186541,-0.707106781186554,-8.65956056235486E-17));
#31663=DIRECTION('center_axis',(0.,-1.,0.));
#31664=DIRECTION('ref_axis',(1.,0.,0.));
#31665=DIRECTION('center_axis',(0.,1.,0.));
#31666=DIRECTION('ref_axis',(0.,0.,1.));
#31667=DIRECTION('center_axis',(0.,-1.,0.));
#31668=DIRECTION('ref_axis',(6.12323399573677E-17,0.,-1.));
#31669=DIRECTION('center_axis',(0.,1.,0.));
#31670=DIRECTION('ref_axis',(1.,0.,0.));
#31671=DIRECTION('center_axis',(0.,1.,0.));
#31672=DIRECTION('ref_axis',(1.,0.,0.));
#31673=DIRECTION('center_axis',(0.,1.,0.));
#31674=DIRECTION('ref_axis',(0.,0.,1.));
#31675=DIRECTION('center_axis',(0.,1.,0.));
#31676=DIRECTION('ref_axis',(1.,0.,0.));
#31677=DIRECTION('center_axis',(0.,1.,0.));
#31678=DIRECTION('ref_axis',(1.,0.,0.));
#31679=DIRECTION('center_axis',(0.,1.,0.));
#31680=DIRECTION('ref_axis',(1.,0.,0.));
#31681=DIRECTION('',(0.,1.,0.));
#31682=DIRECTION('center_axis',(0.,1.,0.));
#31683=DIRECTION('ref_axis',(1.,0.,0.));
#31684=DIRECTION('',(0.707106781186541,-0.707106781186554,-8.65956056235486E-17));
#31685=DIRECTION('center_axis',(0.,-1.,0.));
#31686=DIRECTION('ref_axis',(1.,0.,0.));
#31687=DIRECTION('center_axis',(0.,1.,0.));
#31688=DIRECTION('ref_axis',(1.,0.,0.));
#31689=DIRECTION('center_axis',(0.,1.,0.));
#31690=DIRECTION('ref_axis',(1.,0.,0.));
#31691=DIRECTION('',(0.,1.,0.));
#31692=DIRECTION('center_axis',(0.,1.,0.));
#31693=DIRECTION('ref_axis',(1.,0.,0.));
#31694=DIRECTION('',(0.707106781186547,-0.707106781186547,-8.65956056235493E-17));
#31695=DIRECTION('center_axis',(0.,-1.,0.));
#31696=DIRECTION('ref_axis',(1.,0.,0.));
#31697=DIRECTION('center_axis',(0.,1.,0.));
#31698=DIRECTION('ref_axis',(1.,0.,0.));
#31699=DIRECTION('center_axis',(0.,1.,0.));
#31700=DIRECTION('ref_axis',(1.,0.,0.));
#31701=DIRECTION('',(0.,1.,0.));
#31702=DIRECTION('center_axis',(0.,1.,0.));
#31703=DIRECTION('ref_axis',(1.,0.,0.));
#31704=DIRECTION('',(0.707106781186547,-0.707106781186547,-8.65956056235493E-17));
#31705=DIRECTION('center_axis',(0.,-1.,0.));
#31706=DIRECTION('ref_axis',(1.,0.,0.));
#31707=DIRECTION('center_axis',(0.,1.,0.));
#31708=DIRECTION('ref_axis',(1.,0.,0.));
#31709=DIRECTION('center_axis',(0.,1.,0.));
#31710=DIRECTION('ref_axis',(1.,0.,0.));
#31711=DIRECTION('',(0.,1.,0.));
#31712=DIRECTION('center_axis',(0.,0.,-1.));
#31713=DIRECTION('ref_axis',(1.,0.,0.));
#31714=DIRECTION('center_axis',(0.,0.,-1.));
#31715=DIRECTION('ref_axis',(1.,0.,0.));
#31716=DIRECTION('',(0.707106781186541,-8.65956056235486E-17,0.707106781186554));
#31717=DIRECTION('center_axis',(0.,0.,1.));
#31718=DIRECTION('ref_axis',(1.,0.,0.));
#31719=DIRECTION('',(0.,-1.,0.));
#31720=DIRECTION('center_axis',(0.,0.,1.));
#31721=DIRECTION('ref_axis',(-0.707106781186548,0.707106781186548,0.));
#31722=DIRECTION('',(-1.,0.,0.));
#31723=DIRECTION('center_axis',(0.,0.,1.));
#31724=DIRECTION('ref_axis',(0.707106781186549,0.707106781186547,0.));
#31725=DIRECTION('',(0.,1.,0.));
#31726=DIRECTION('center_axis',(0.,0.,1.));
#31727=DIRECTION('ref_axis',(0.707106781186548,-0.707106781186548,0.));
#31728=DIRECTION('',(1.,0.,0.));
#31729=DIRECTION('center_axis',(0.,0.,1.));
#31730=DIRECTION('ref_axis',(-0.707106781186549,-0.707106781186547,0.));
#31731=DIRECTION('center_axis',(0.,0.,-1.));
#31732=DIRECTION('ref_axis',(1.,0.,0.));
#31733=DIRECTION('center_axis',(0.,0.,-1.));
#31734=DIRECTION('ref_axis',(1.,0.,0.));
#31735=DIRECTION('',(0.707106781186541,-8.65956056235486E-17,0.707106781186554));
#31736=DIRECTION('center_axis',(0.,-1.,0.));
#31737=DIRECTION('ref_axis',(0.,0.,1.));
#31738=DIRECTION('center_axis',(0.,1.,0.));
#31739=DIRECTION('ref_axis',(0.,0.,1.));
#31740=DIRECTION('center_axis',(1.,0.,-1.22464679914735E-16));
#31741=DIRECTION('ref_axis',(-1.22464679914735E-16,0.,-1.));
#31742=DIRECTION('center_axis',(0.,-1.,0.));
#31743=DIRECTION('ref_axis',(0.,0.,1.));
#31744=DIRECTION('center_axis',(0.,1.,0.));
#31745=DIRECTION('ref_axis',(0.,0.,1.));
#31746=DIRECTION('',(0.,-1.,0.));
#31747=DIRECTION('center_axis',(0.,-1.,0.));
#31748=DIRECTION('ref_axis',(1.22464679914735E-16,0.,1.));
#31749=DIRECTION('center_axis',(0.,1.,0.));
#31750=DIRECTION('ref_axis',(0.,0.,1.));
#31751=DIRECTION('center_axis',(0.,-1.,0.));
#31752=DIRECTION('ref_axis',(1.,0.,0.));
#31753=DIRECTION('center_axis',(0.,-1.,0.));
#31754=DIRECTION('ref_axis',(1.,0.,0.));
#31755=DIRECTION('center_axis',(0.,-1.,0.));
#31756=DIRECTION('ref_axis',(1.,0.,0.));
#31757=DIRECTION('center_axis',(0.,-1.,0.));
#31758=DIRECTION('ref_axis',(1.,0.,0.));
#31759=DIRECTION('center_axis',(0.,1.,0.));
#31760=DIRECTION('ref_axis',(1.,0.,0.));
#31761=DIRECTION('center_axis',(0.,1.,0.));
#31762=DIRECTION('ref_axis',(1.22464679914735E-16,0.,1.));
#31763=DIRECTION('center_axis',(-1.,0.,0.));
#31764=DIRECTION('ref_axis',(0.,0.,-1.));
#31765=DIRECTION('center_axis',(0.,1.,0.));
#31766=DIRECTION('ref_axis',(1.22464679914735E-16,0.,1.));
#31767=DIRECTION('center_axis',(0.,-1.,0.));
#31768=DIRECTION('ref_axis',(0.,0.,-1.));
#31769=DIRECTION('center_axis',(0.,1.,0.));
#31770=DIRECTION('ref_axis',(1.,0.,0.));
#31771=DIRECTION('center_axis',(0.,1.,0.));
#31772=DIRECTION('ref_axis',(1.,0.,0.));
#31773=DIRECTION('center_axis',(0.,1.,0.));
#31774=DIRECTION('ref_axis',(1.,0.,0.));
#31775=DIRECTION('center_axis',(0.,1.,0.));
#31776=DIRECTION('ref_axis',(1.,0.,0.));
#31777=DIRECTION('center_axis',(0.,1.,0.));
#31778=DIRECTION('ref_axis',(1.,0.,0.));
#31779=DIRECTION('center_axis',(0.,1.,0.));
#31780=DIRECTION('ref_axis',(0.,0.,1.));
#31781=DIRECTION('center_axis',(0.,-1.,0.));
#31782=DIRECTION('ref_axis',(-3.06161699786838E-17,0.,-1.));
#31783=DIRECTION('center_axis',(-1.,0.,1.22464679914735E-16));
#31784=DIRECTION('ref_axis',(-1.22464679914735E-16,0.,-1.));
#31785=DIRECTION('center_axis',(0.,1.,0.));
#31786=DIRECTION('ref_axis',(-3.06161699786838E-17,0.,-1.));
#31787=DIRECTION('center_axis',(0.,1.,0.));
#31788=DIRECTION('ref_axis',(0.,0.,1.));
#31789=DIRECTION('',(1.20086498579063E-16,-0.196116135138187,0.98058067569092));
#31790=DIRECTION('center_axis',(0.,-1.,0.));
#31791=DIRECTION('ref_axis',(-3.06161699786838E-17,0.,-1.));
#31792=DIRECTION('center_axis',(0.,1.,0.));
#31793=DIRECTION('ref_axis',(0.,0.,1.));
#31794=DIRECTION('center_axis',(0.,1.,0.));
#31795=DIRECTION('ref_axis',(1.,0.,0.));
#31796=DIRECTION('',(8.65956056235501E-17,-0.707106781186541,0.707106781186554));
#31797=DIRECTION('center_axis',(0.,1.,0.));
#31798=DIRECTION('ref_axis',(0.,0.,1.));
#31799=DIRECTION('center_axis',(-1.,0.,1.22464679914735E-16));
#31800=DIRECTION('ref_axis',(-1.22464679914735E-16,0.,-1.));
#31801=DIRECTION('center_axis',(0.,1.,0.));
#31802=DIRECTION('ref_axis',(-3.06161699786838E-17,0.,-1.));
#31803=DIRECTION('center_axis',(0.,1.,0.));
#31804=DIRECTION('ref_axis',(0.,0.,1.));
#31805=DIRECTION('',(1.2221746482687E-16,-0.0635079031754479,0.997981335614178));
#31806=DIRECTION('center_axis',(0.,1.,0.));
#31807=DIRECTION('ref_axis',(0.,0.,1.));
#31808=DIRECTION('center_axis',(0.,-1.,0.));
#31809=DIRECTION('ref_axis',(-1.,0.,-1.11022302462516E-16));
#31810=DIRECTION('center_axis',(0.,-1.,0.));
#31811=DIRECTION('ref_axis',(9.18485099360515E-17,0.,1.));
#31812=DIRECTION('center_axis',(0.,-1.,0.));
#31813=DIRECTION('ref_axis',(1.,0.,0.));
#31814=DIRECTION('center_axis',(0.,1.,0.));
#31815=DIRECTION('ref_axis',(0.,0.,1.));
#31816=DIRECTION('center_axis',(0.,1.,0.));
#31817=DIRECTION('ref_axis',(0.,0.,1.));
#31818=DIRECTION('center_axis',(0.,1.,0.));
#31819=DIRECTION('ref_axis',(1.,0.,0.));
#31820=DIRECTION('center_axis',(0.,-1.,0.));
#31821=DIRECTION('ref_axis',(0.,0.,-1.));
#31822=DIRECTION('',(0.,0.,1.));
#31823=DIRECTION('center_axis',(0.,1.,0.));
#31824=DIRECTION('ref_axis',(0.,0.,1.));
#31825=DIRECTION('center_axis',(0.,1.,0.));
#31826=DIRECTION('ref_axis',(6.12323399573677E-17,0.,1.));
#31827=DIRECTION('center_axis',(0.,-1.,0.));
#31828=DIRECTION('ref_axis',(0.,0.,-1.));
#31829=DIRECTION('',(-1.,0.,0.));
#31830=DIRECTION('center_axis',(0.,1.,0.));
#31831=DIRECTION('ref_axis',(0.,0.,1.));
#31832=DIRECTION('center_axis',(0.,1.,0.));
#31833=DIRECTION('ref_axis',(-1.,0.,-1.22464679914735E-16));
#31834=DIRECTION('center_axis',(0.,-1.,0.));
#31835=DIRECTION('ref_axis',(0.,0.,-1.));
#31836=DIRECTION('center_axis',(0.,-1.,0.));
#31837=DIRECTION('ref_axis',(-0.707106781186551,0.,-0.707106781186544));
#31838=DIRECTION('center_axis',(0.,-1.,0.));
#31839=DIRECTION('ref_axis',(-1.,0.,0.));
#31840=DIRECTION('center_axis',(0.,1.,0.));
#31841=DIRECTION('ref_axis',(0.,0.,-1.));
#31842=DIRECTION('',(0.,1.,0.));
#31843=DIRECTION('center_axis',(-1.,0.,0.));
#31844=DIRECTION('ref_axis',(0.,0.,-1.));
#31845=DIRECTION('center_axis',(0.,0.,-1.));
#31846=DIRECTION('ref_axis',(-0.707106781186549,-0.707106781186546,0.));
#31847=DIRECTION('center_axis',(1.,0.,0.));
#31848=DIRECTION('ref_axis',(0.,-0.707106781186554,-0.707106781186541));
#31849=DIRECTION('center_axis',(-1.,-4.44089209850056E-15,0.));
#31850=DIRECTION('ref_axis',(0.,0.,-1.));
#31851=DIRECTION('',(-1.,0.,0.));
#31852=DIRECTION('center_axis',(0.,-1.,0.));
#31853=DIRECTION('ref_axis',(0.,0.,-1.));
#31854=DIRECTION('center_axis',(0.,0.,-1.));
#31855=DIRECTION('ref_axis',(0.707106781186548,-0.707106781186548,0.));
#31856=DIRECTION('center_axis',(0.,1.,0.));
#31857=DIRECTION('ref_axis',(0.707106781186551,0.,-0.707106781186544));
#31858=DIRECTION('center_axis',(0.,-1.,0.));
#31859=DIRECTION('ref_axis',(0.,0.,-1.));
#31860=DIRECTION('',(0.,-1.,0.));
#31861=DIRECTION('center_axis',(1.,0.,0.));
#31862=DIRECTION('ref_axis',(0.,0.,-1.));
#31863=DIRECTION('center_axis',(0.,0.,-1.));
#31864=DIRECTION('ref_axis',(0.707106781186549,0.707106781186546,0.));
#31865=DIRECTION('center_axis',(-1.,0.,0.));
#31866=DIRECTION('ref_axis',(0.,0.707106781186554,-0.707106781186541));
#31867=DIRECTION('center_axis',(1.,4.44089209850056E-15,0.));
#31868=DIRECTION('ref_axis',(0.,0.,-1.));
#31869=DIRECTION('',(1.,0.,0.));
#31870=DIRECTION('center_axis',(0.,0.,-1.));
#31871=DIRECTION('ref_axis',(-0.707106781186548,0.707106781186548,0.));
#31872=DIRECTION('center_axis',(0.,0.,1.));
#31873=DIRECTION('ref_axis',(1.,0.,0.));
#31874=DIRECTION('',(0.,0.,1.));
#31875=DIRECTION('',(0.,0.,1.));
#31876=DIRECTION('center_axis',(0.,1.,0.));
#31877=DIRECTION('ref_axis',(-1.,0.,0.));
#31878=DIRECTION('',(0.,0.,1.));
#31879=DIRECTION('center_axis',(0.,0.,1.));
#31880=DIRECTION('ref_axis',(0.,1.,0.));
#31881=DIRECTION('',(0.,0.,1.));
#31882=DIRECTION('center_axis',(-1.,0.,0.));
#31883=DIRECTION('ref_axis',(0.,-1.,0.));
#31884=DIRECTION('',(0.,0.,1.));
#31885=DIRECTION('center_axis',(0.,1.,0.));
#31886=DIRECTION('ref_axis',(0.,0.,1.));
#31887=DIRECTION('center_axis',(-1.,0.,1.22464679914735E-16));
#31888=DIRECTION('ref_axis',(-1.22464679914735E-16,0.,-1.));
#31889=DIRECTION('center_axis',(0.,1.,0.));
#31890=DIRECTION('ref_axis',(6.12323399573677E-17,0.,-1.));
#31891=DIRECTION('center_axis',(0.,1.,0.));
#31892=DIRECTION('ref_axis',(0.,0.,1.));
#31893=DIRECTION('',(0.,-1.,0.));
#31894=DIRECTION('',(0.,1.,0.));
#31895=DIRECTION('center_axis',(0.,1.,0.));
#31896=DIRECTION('ref_axis',(0.,0.,1.));
#31897=DIRECTION('center_axis',(0.,-1.,0.));
#31898=DIRECTION('ref_axis',(0.,0.,1.));
#31899=DIRECTION('center_axis',(-1.,0.,1.22464679914735E-16));
#31900=DIRECTION('ref_axis',(-1.22464679914735E-16,0.,-1.));
#31901=DIRECTION('center_axis',(0.,1.,0.));
#31902=DIRECTION('ref_axis',(0.,0.,1.));
#31903=DIRECTION('center_axis',(0.,-1.,0.));
#31904=DIRECTION('ref_axis',(0.,0.,1.));
#31905=DIRECTION('center_axis',(0.,-1.,0.));
#31906=DIRECTION('ref_axis',(0.,0.,1.));
#31907=DIRECTION('center_axis',(0.,-1.,0.));
#31908=DIRECTION('ref_axis',(0.,0.,1.));
#31909=DIRECTION('center_axis',(0.,1.,0.));
#31910=DIRECTION('ref_axis',(1.,0.,0.));
#31911=DIRECTION('',(0.,0.,-1.));
#31912=DIRECTION('center_axis',(0.,1.,0.));
#31913=DIRECTION('ref_axis',(2.96059473233374E-15,0.,1.));
#31914=DIRECTION('',(1.,0.,0.));
#31915=DIRECTION('center_axis',(0.,1.,0.));
#31916=DIRECTION('ref_axis',(1.,0.,0.));
#31917=DIRECTION('',(-1.,0.,0.));
#31918=DIRECTION('center_axis',(0.,1.,0.));
#31919=DIRECTION('ref_axis',(1.,0.,-2.96059473233374E-15));
#31920=DIRECTION('',(0.,0.,-1.));
#31921=DIRECTION('center_axis',(0.,1.,0.));
#31922=DIRECTION('ref_axis',(1.,0.,0.));
#31923=DIRECTION('',(-1.,0.,0.));
#31924=DIRECTION('center_axis',(0.,1.,0.));
#31925=DIRECTION('ref_axis',(1.,0.,0.));
#31926=DIRECTION('',(1.,0.,0.));
#31927=DIRECTION('center_axis',(0.,1.,0.));
#31928=DIRECTION('ref_axis',(-1.,0.,2.96059473233374E-15));
#31929=DIRECTION('center_axis',(0.,1.,0.));
#31930=DIRECTION('ref_axis',(0.,0.,1.));
#31931=DIRECTION('center_axis',(0.,-1.,0.));
#31932=DIRECTION('ref_axis',(0.,0.,1.));
#31933=DIRECTION('',(0.,-1.,0.));
#31934=DIRECTION('center_axis',(0.,-1.,0.));
#31935=DIRECTION('ref_axis',(0.,0.,-1.));
#31936=DIRECTION('center_axis',(-1.,0.,-1.22464679914735E-16));
#31937=DIRECTION('ref_axis',(-1.22464679914735E-16,0.,1.));
#31938=DIRECTION('center_axis',(0.,-1.,0.));
#31939=DIRECTION('ref_axis',(0.,0.,1.));
#31940=DIRECTION('center_axis',(0.,-1.,0.));
#31941=DIRECTION('ref_axis',(0.,0.,1.));
#31942=DIRECTION('center_axis',(0.,1.,0.));
#31943=DIRECTION('ref_axis',(0.,0.,1.));
#31944=DIRECTION('center_axis',(0.,1.,0.));
#31945=DIRECTION('ref_axis',(1.,0.,0.));
#31946=DIRECTION('',(0.,1.,0.));
#31947=DIRECTION('center_axis',(0.,1.,0.));
#31948=DIRECTION('ref_axis',(0.,0.,1.));
#31949=DIRECTION('center_axis',(-1.,0.,1.22464679914735E-16));
#31950=DIRECTION('ref_axis',(-1.22464679914735E-16,0.,-1.));
#31951=DIRECTION('center_axis',(0.,1.,0.));
#31952=DIRECTION('ref_axis',(0.,0.,1.));
#31953=DIRECTION('center_axis',(0.,-1.,0.));
#31954=DIRECTION('ref_axis',(0.,0.,-1.));
#31955=DIRECTION('center_axis',(0.,1.,0.));
#31956=DIRECTION('ref_axis',(0.707106781186546,0.,-0.707106781186549));
#31957=DIRECTION('center_axis',(0.,1.,0.));
#31958=DIRECTION('ref_axis',(1.,0.,0.));
#31959=DIRECTION('',(0.,1.,0.));
#31960=DIRECTION('center_axis',(0.,-1.,0.));
#31961=DIRECTION('ref_axis',(0.,0.,-1.));
#31962=DIRECTION('',(0.,-1.,0.));
#31963=DIRECTION('center_axis',(-1.,0.,0.));
#31964=DIRECTION('ref_axis',(0.,0.,1.));
#31965=DIRECTION('center_axis',(0.,2.22044604925032E-15,1.));
#31966=DIRECTION('ref_axis',(0.,-1.,2.22044604925032E-15));
#31967=DIRECTION('center_axis',(1.,0.,0.));
#31968=DIRECTION('ref_axis',(0.,0.707106781186548,0.707106781186547));
#31969=DIRECTION('center_axis',(-1.,0.,0.));
#31970=DIRECTION('ref_axis',(0.,0.707106781186548,0.707106781186547));
#31971=DIRECTION('center_axis',(0.,0.,-1.));
#31972=DIRECTION('ref_axis',(0.707106781186541,-0.707106781186554,0.));
#31973=DIRECTION('center_axis',(0.,-2.22044604925032E-15,1.));
#31974=DIRECTION('ref_axis',(0.,-1.,-2.22044604925032E-15));
#31975=DIRECTION('',(0.,0.,1.));
#31976=DIRECTION('',(0.,0.,-1.));
#31977=DIRECTION('center_axis',(-1.,0.,0.));
#31978=DIRECTION('ref_axis',(0.,0.,1.));
#31979=DIRECTION('center_axis',(0.,1.,0.));
#31980=DIRECTION('ref_axis',(0.,0.,1.));
#31981=DIRECTION('center_axis',(1.,0.,0.));
#31982=DIRECTION('ref_axis',(0.,0.707106781186548,-0.707106781186547));
#31983=DIRECTION('center_axis',(-1.,0.,0.));
#31984=DIRECTION('ref_axis',(0.,0.707106781186548,-0.707106781186547));
#31985=DIRECTION('center_axis',(0.,-1.,0.));
#31986=DIRECTION('ref_axis',(0.707106781186546,0.,0.707106781186549));
#31987=DIRECTION('center_axis',(0.,1.,0.));
#31988=DIRECTION('ref_axis',(0.,0.,1.));
#31989=DIRECTION('',(0.,1.,0.));
#31990=DIRECTION('',(0.,-1.,0.));
#31991=DIRECTION('center_axis',(-1.,0.,0.));
#31992=DIRECTION('ref_axis',(0.,0.,1.));
#31993=DIRECTION('center_axis',(0.,2.22044604925032E-15,-1.));
#31994=DIRECTION('ref_axis',(0.,1.,2.22044604925032E-15));
#31995=DIRECTION('center_axis',(1.,0.,0.));
#31996=DIRECTION('ref_axis',(0.,-0.707106781186547,-0.707106781186548));
#31997=DIRECTION('center_axis',(-1.,0.,0.));
#31998=DIRECTION('ref_axis',(0.,-0.707106781186547,-0.707106781186548));
#31999=DIRECTION('center_axis',(0.,0.,1.));
#32000=DIRECTION('ref_axis',(0.707106781186548,0.707106781186548,0.));
#32001=DIRECTION('center_axis',(0.,0.,-1.));
#32002=DIRECTION('ref_axis',(0.,1.,0.));
#32003=DIRECTION('',(0.,0.,-1.));
#32004=DIRECTION('',(0.,0.,1.));
#32005=DIRECTION('center_axis',(-1.,0.,0.));
#32006=DIRECTION('ref_axis',(0.,0.,1.));
#32007=DIRECTION('center_axis',(1.,0.,0.));
#32008=DIRECTION('ref_axis',(0.,-0.707106781186548,0.707106781186548));
#32009=DIRECTION('center_axis',(-1.,0.,0.));
#32010=DIRECTION('ref_axis',(0.,-0.707106781186548,0.707106781186548));
#32011=DIRECTION('center_axis',(-1.,0.,0.));
#32012=DIRECTION('ref_axis',(0.,0.,-1.));
#32013=DIRECTION('',(-1.,0.,0.));
#32014=DIRECTION('center_axis',(1.,0.,0.));
#32015=DIRECTION('ref_axis',(0.,0.707106781186548,-0.707106781186547));
#32016=DIRECTION('',(-1.,0.,0.));
#32017=DIRECTION('center_axis',(0.,1.,0.));
#32018=DIRECTION('ref_axis',(0.,0.,-1.));
#32019=DIRECTION('',(-1.,0.,0.));
#32020=DIRECTION('',(0.,0.,1.));
#32021=DIRECTION('center_axis',(-1.,0.,0.));
#32022=DIRECTION('ref_axis',(0.,1.,-2.22044604925032E-15));
#32023=DIRECTION('',(-1.,0.,0.));
#32024=DIRECTION('center_axis',(1.,0.,0.));
#32025=DIRECTION('ref_axis',(0.,0.707106781186548,0.707106781186547));
#32026=DIRECTION('center_axis',(0.,0.,1.));
#32027=DIRECTION('ref_axis',(0.,1.,0.));
#32028=DIRECTION('',(-1.,0.,0.));
#32029=DIRECTION('',(0.,-1.,0.));
#32030=DIRECTION('center_axis',(1.,0.,0.));
#32031=DIRECTION('ref_axis',(0.,0.,-1.));
#32032=DIRECTION('',(0.,0.,1.));
#32033=DIRECTION('',(0.,1.,0.));
#32034=DIRECTION('',(0.,1.,0.));
#32035=DIRECTION('center_axis',(0.,-1.,0.));
#32036=DIRECTION('ref_axis',(-0.707106781186546,0.,-0.707106781186549));
#32037=DIRECTION('center_axis',(0.,-1.,0.));
#32038=DIRECTION('ref_axis',(-1.,0.,0.));
#32039=DIRECTION('center_axis',(0.,1.,0.));
#32040=DIRECTION('ref_axis',(0.,0.,-1.));
#32041=DIRECTION('',(0.,1.,0.));
#32042=DIRECTION('center_axis',(1.,0.,0.));
#32043=DIRECTION('ref_axis',(0.,0.,-1.));
#32044=DIRECTION('center_axis',(0.,2.22044604925032E-15,1.));
#32045=DIRECTION('ref_axis',(0.,1.,-2.22044604925032E-15));
#32046=DIRECTION('center_axis',(-1.,0.,0.));
#32047=DIRECTION('ref_axis',(0.,-0.707106781186548,0.707106781186548));
#32048=DIRECTION('center_axis',(1.,0.,0.));
#32049=DIRECTION('ref_axis',(0.,-0.707106781186548,0.707106781186548));
#32050=DIRECTION('center_axis',(0.,0.,-1.));
#32051=DIRECTION('ref_axis',(-0.707106781186548,0.707106781186548,0.));
#32052=DIRECTION('center_axis',(0.,-2.22044604925032E-15,1.));
#32053=DIRECTION('ref_axis',(0.,1.,2.22044604925032E-15));
#32054=DIRECTION('',(0.,0.,1.));
#32055=DIRECTION('',(0.,0.,-1.));
#32056=DIRECTION('center_axis',(1.,0.,0.));
#32057=DIRECTION('ref_axis',(0.,0.,-1.));
#32058=DIRECTION('center_axis',(0.,-1.,0.));
#32059=DIRECTION('ref_axis',(0.,0.,1.));
#32060=DIRECTION('center_axis',(-1.,0.,0.));
#32061=DIRECTION('ref_axis',(0.,-0.707106781186547,-0.707106781186548));
#32062=DIRECTION('center_axis',(1.,0.,0.));
#32063=DIRECTION('ref_axis',(0.,-0.707106781186547,-0.707106781186548));
#32064=DIRECTION('center_axis',(0.,1.,0.));
#32065=DIRECTION('ref_axis',(-0.707106781186546,0.,0.707106781186549));
#32066=DIRECTION('center_axis',(0.,-1.,0.));
#32067=DIRECTION('ref_axis',(0.,0.,1.));
#32068=DIRECTION('',(0.,-1.,0.));
#32069=DIRECTION('',(0.,1.,0.));
#32070=DIRECTION('center_axis',(1.,0.,0.));
#32071=DIRECTION('ref_axis',(0.,0.,-1.));
#32072=DIRECTION('center_axis',(0.,2.22044604925032E-15,-1.));
#32073=DIRECTION('ref_axis',(0.,-1.,-2.22044604925032E-15));
#32074=DIRECTION('center_axis',(-1.,0.,0.));
#32075=DIRECTION('ref_axis',(0.,0.707106781186548,-0.707106781186547));
#32076=DIRECTION('center_axis',(0.,0.,1.));
#32077=DIRECTION('ref_axis',(-0.707106781186541,-0.707106781186554,0.));
#32078=DIRECTION('center_axis',(0.,0.,-1.));
#32079=DIRECTION('ref_axis',(0.,-1.,0.));
#32080=DIRECTION('',(0.,0.,-1.));
#32081=DIRECTION('center_axis',(1.,0.,0.));
#32082=DIRECTION('ref_axis',(0.,0.,-1.));
#32083=DIRECTION('center_axis',(-1.,0.,0.));
#32084=DIRECTION('ref_axis',(0.,0.707106781186548,0.707106781186547));
#32085=DIRECTION('center_axis',(-1.,0.,0.));
#32086=DIRECTION('ref_axis',(0.,-1.,-1.48029736616687E-15));
#32087=DIRECTION('',(-1.,0.,0.));
#32088=DIRECTION('',(-1.,0.,0.));
#32089=DIRECTION('center_axis',(0.,-1.,0.));
#32090=DIRECTION('ref_axis',(0.,0.,1.));
#32091=DIRECTION('',(-1.,0.,0.));
#32092=DIRECTION('center_axis',(-1.,0.,0.));
#32093=DIRECTION('ref_axis',(0.,0.,1.));
#32094=DIRECTION('center_axis',(1.,0.,0.));
#32095=DIRECTION('ref_axis',(0.,0.,-1.));
#32096=DIRECTION('',(0.,1.,0.));
#32097=DIRECTION('',(0.,1.,0.));
#32098=DIRECTION('center_axis',(0.,0.,-1.));
#32099=DIRECTION('ref_axis',(-0.707106781186551,-0.707106781186544,0.));
#32100=DIRECTION('center_axis',(4.44089209850062E-15,0.,-1.));
#32101=DIRECTION('ref_axis',(0.,-1.,0.));
#32102=DIRECTION('center_axis',(0.,0.,1.));
#32103=DIRECTION('ref_axis',(-1.,0.,0.));
#32104=DIRECTION('',(0.,0.,1.));
#32105=DIRECTION('center_axis',(0.,1.,0.));
#32106=DIRECTION('ref_axis',(0.,0.,1.));
#32107=DIRECTION('center_axis',(-1.,0.,0.));
#32108=DIRECTION('ref_axis',(0.,0.,-1.));
#32109=DIRECTION('center_axis',(0.,1.,0.));
#32110=DIRECTION('ref_axis',(-0.707106781186548,0.,-0.707106781186548));
#32111=DIRECTION('center_axis',(0.,-1.,0.));
#32112=DIRECTION('ref_axis',(-0.707106781186548,0.,-0.707106781186548));
#32113=DIRECTION('center_axis',(1.,0.,0.));
#32114=DIRECTION('ref_axis',(0.,-0.707106781186544,-0.707106781186551));
#32115=DIRECTION('center_axis',(-1.,0.,0.));
#32116=DIRECTION('ref_axis',(0.,0.,-1.));
#32117=DIRECTION('',(-1.,0.,0.));
#32118=DIRECTION('',(1.,0.,0.));
#32119=DIRECTION('center_axis',(0.,1.,0.));
#32120=DIRECTION('ref_axis',(0.,0.,1.));
#32121=DIRECTION('center_axis',(0.,0.,-1.));
#32122=DIRECTION('ref_axis',(1.,0.,0.));
#32123=DIRECTION('center_axis',(0.,1.,0.));
#32124=DIRECTION('ref_axis',(0.707106781186548,0.,-0.707106781186548));
#32125=DIRECTION('center_axis',(0.,-1.,0.));
#32126=DIRECTION('ref_axis',(0.707106781186548,0.,-0.707106781186548));
#32127=DIRECTION('center_axis',(0.,0.,1.));
#32128=DIRECTION('ref_axis',(0.707106781186551,-0.707106781186544,0.));
#32129=DIRECTION('center_axis',(0.,0.,-1.));
#32130=DIRECTION('ref_axis',(1.,0.,0.));
#32131=DIRECTION('',(0.,0.,-1.));
#32132=DIRECTION('center_axis',(0.,1.,0.));
#32133=DIRECTION('ref_axis',(0.,0.,1.));
#32134=DIRECTION('center_axis',(1.,0.,0.));
#32135=DIRECTION('ref_axis',(0.,0.,1.));
#32136=DIRECTION('center_axis',(0.,1.,0.));
#32137=DIRECTION('ref_axis',(0.707106781186548,0.,0.707106781186548));
#32138=DIRECTION('center_axis',(0.,-1.,0.));
#32139=DIRECTION('ref_axis',(0.707106781186548,0.,0.707106781186548));
#32140=DIRECTION('center_axis',(-1.,0.,0.));
#32141=DIRECTION('ref_axis',(0.,-0.707106781186544,0.707106781186551));
#32142=DIRECTION('center_axis',(1.,0.,0.));
#32143=DIRECTION('ref_axis',(0.,0.,1.));
#32144=DIRECTION('',(1.,0.,0.));
#32145=DIRECTION('',(-1.,0.,0.));
#32146=DIRECTION('center_axis',(0.,1.,0.));
#32147=DIRECTION('ref_axis',(0.,0.,1.));
#32148=DIRECTION('center_axis',(0.,-1.,0.));
#32149=DIRECTION('ref_axis',(-0.707106781186548,0.,0.707106781186548));
#32150=DIRECTION('center_axis',(0.,1.,0.));
#32151=DIRECTION('ref_axis',(-0.707106781186548,0.,0.707106781186548));
#32152=DIRECTION('center_axis',(0.,1.,0.));
#32153=DIRECTION('ref_axis',(1.,0.,0.));
#32154=DIRECTION('',(0.,1.,0.));
#32155=DIRECTION('center_axis',(0.,0.,-1.));
#32156=DIRECTION('ref_axis',(-1.,0.,0.));
#32157=DIRECTION('',(0.,1.,0.));
#32158=DIRECTION('center_axis',(0.,0.,1.));
#32159=DIRECTION('ref_axis',(4.44089209850064E-15,1.,0.));
#32160=DIRECTION('',(0.,-1.,0.));
#32161=DIRECTION('center_axis',(0.,0.,1.));
#32162=DIRECTION('ref_axis',(-1.,0.,0.));
#32163=DIRECTION('',(1.,0.,0.));
#32164=DIRECTION('center_axis',(0.,0.,1.));
#32165=DIRECTION('ref_axis',(-4.44089209850064E-15,-1.,0.));
#32166=DIRECTION('',(0.,1.,0.));
#32167=DIRECTION('center_axis',(0.,0.,1.));
#32168=DIRECTION('ref_axis',(1.,0.,0.));
#32169=DIRECTION('center_axis',(0.,1.,0.));
#32170=DIRECTION('ref_axis',(0.,0.,-1.));
#32171=DIRECTION('center_axis',(0.,1.,0.));
#32172=DIRECTION('ref_axis',(1.,0.,0.));
#32173=DIRECTION('center_axis',(0.,-1.,0.));
#32174=DIRECTION('ref_axis',(0.,0.,1.));
#32175=DIRECTION('center_axis',(0.,0.,1.));
#32176=DIRECTION('ref_axis',(-0.707106781186541,-0.707106781186554,0.));
#32177=DIRECTION('center_axis',(0.,0.,1.));
#32178=DIRECTION('ref_axis',(-1.,0.,0.));
#32179=DIRECTION('',(0.,0.,1.));
#32180=DIRECTION('center_axis',(0.,-2.22044604925032E-15,-1.));
#32181=DIRECTION('ref_axis',(0.,-1.,2.22044604925032E-15));
#32182=DIRECTION('center_axis',(1.,0.,0.));
#32183=DIRECTION('ref_axis',(0.,0.,-1.));
#32184=DIRECTION('center_axis',(0.,1.,0.));
#32185=DIRECTION('ref_axis',(0.,0.,-1.));
#32186=DIRECTION('center_axis',(1.,0.,0.));
#32187=DIRECTION('ref_axis',(0.,0.707106781186548,0.707106781186547));
#32188=DIRECTION('center_axis',(0.,-1.,0.));
#32189=DIRECTION('ref_axis',(-0.707106781186546,0.,-0.707106781186549));
#32190=DIRECTION('center_axis',(0.,1.,0.));
#32191=DIRECTION('ref_axis',(0.,0.,-1.));
#32192=DIRECTION('',(0.,-1.,0.));
#32193=DIRECTION('center_axis',(1.,0.,0.));
#32194=DIRECTION('ref_axis',(0.,0.,-1.));
#32195=DIRECTION('center_axis',(0.,2.22044604925032E-15,1.));
#32196=DIRECTION('ref_axis',(0.,1.,-2.22044604925032E-15));
#32197=DIRECTION('center_axis',(1.,0.,0.));
#32198=DIRECTION('ref_axis',(0.,-0.707106781186548,0.707106781186548));
#32199=DIRECTION('center_axis',(0.,0.,-1.));
#32200=DIRECTION('ref_axis',(-0.707106781186548,0.707106781186548,0.));
#32201=DIRECTION('center_axis',(0.,0.,1.));
#32202=DIRECTION('ref_axis',(0.,1.,0.));
#32203=DIRECTION('',(0.,0.,-1.));
#32204=DIRECTION('center_axis',(1.,0.,0.));
#32205=DIRECTION('ref_axis',(0.,0.,-1.));
#32206=DIRECTION('center_axis',(0.,-1.,0.));
#32207=DIRECTION('ref_axis',(0.,0.,1.));
#32208=DIRECTION('center_axis',(1.,0.,0.));
#32209=DIRECTION('ref_axis',(0.,-0.707106781186547,-0.707106781186548));
#32210=DIRECTION('center_axis',(0.,1.,0.));
#32211=DIRECTION('ref_axis',(-0.707106781186546,0.,0.707106781186549));
#32212=DIRECTION('center_axis',(0.,-1.,0.));
#32213=DIRECTION('ref_axis',(0.,0.,1.));
#32214=DIRECTION('',(0.,1.,0.));
#32215=DIRECTION('center_axis',(1.,0.,0.));
#32216=DIRECTION('ref_axis',(0.,0.,-1.));
#32217=DIRECTION('center_axis',(1.,0.,0.));
#32218=DIRECTION('ref_axis',(0.,0.707106781186548,-0.707106781186547));
#32219=DIRECTION('center_axis',(1.,0.,0.));
#32220=DIRECTION('ref_axis',(0.,0.,1.));
#32221=DIRECTION('',(1.,0.,0.));
#32222=DIRECTION('center_axis',(-1.,0.,0.));
#32223=DIRECTION('ref_axis',(0.,-0.707106781186548,0.707106781186548));
#32224=DIRECTION('',(1.,0.,0.));
#32225=DIRECTION('center_axis',(0.,0.,1.));
#32226=DIRECTION('ref_axis',(0.,-1.,0.));
#32227=DIRECTION('',(1.,0.,0.));
#32228=DIRECTION('',(0.,1.,0.));
#32229=DIRECTION('center_axis',(1.,0.,0.));
#32230=DIRECTION('ref_axis',(0.,1.,-2.22044604925032E-15));
#32231=DIRECTION('',(1.,0.,0.));
#32232=DIRECTION('center_axis',(-1.,0.,0.));
#32233=DIRECTION('ref_axis',(0.,0.707106781186548,0.707106781186547));
#32234=DIRECTION('center_axis',(0.,1.,0.));
#32235=DIRECTION('ref_axis',(0.,0.,1.));
#32236=DIRECTION('',(1.,0.,0.));
#32237=DIRECTION('',(0.,0.,-1.));
#32238=DIRECTION('center_axis',(0.,0.,-1.));
#32239=DIRECTION('ref_axis',(0.707106781186541,-0.707106781186554,0.));
#32240=DIRECTION('center_axis',(0.,2.22044604925032E-15,-1.));
#32241=DIRECTION('ref_axis',(1.,0.,0.));
#32242=DIRECTION('center_axis',(0.,0.,1.));
#32243=DIRECTION('ref_axis',(0.,-1.,0.));
#32244=DIRECTION('center_axis',(-1.,0.,0.));
#32245=DIRECTION('ref_axis',(0.,0.,1.));
#32246=DIRECTION('center_axis',(0.,1.,0.));
#32247=DIRECTION('ref_axis',(0.,0.,1.));
#32248=DIRECTION('center_axis',(-1.,0.,0.));
#32249=DIRECTION('ref_axis',(0.,0.707106781186548,-0.707106781186547));
#32250=DIRECTION('center_axis',(0.,-1.,0.));
#32251=DIRECTION('ref_axis',(0.707106781186546,0.,0.707106781186549));
#32252=DIRECTION('center_axis',(0.,1.,0.));
#32253=DIRECTION('ref_axis',(0.,0.,1.));
#32254=DIRECTION('',(0.,-1.,0.));
#32255=DIRECTION('center_axis',(-1.,0.,0.));
#32256=DIRECTION('ref_axis',(0.,0.,1.));
#32257=DIRECTION('center_axis',(0.,2.22044604925032E-15,-1.));
#32258=DIRECTION('ref_axis',(0.,1.,2.22044604925032E-15));
#32259=DIRECTION('center_axis',(-1.,0.,0.));
#32260=DIRECTION('ref_axis',(0.,-0.707106781186547,-0.707106781186548));
#32261=DIRECTION('center_axis',(0.,0.,1.));
#32262=DIRECTION('ref_axis',(0.707106781186548,0.707106781186548,0.));
#32263=DIRECTION('center_axis',(0.,-2.22044604925032E-15,-1.));
#32264=DIRECTION('ref_axis',(0.,1.,-2.22044604925032E-15));
#32265=DIRECTION('',(0.,0.,1.));
#32266=DIRECTION('center_axis',(-1.,0.,0.));
#32267=DIRECTION('ref_axis',(0.,0.,1.));
#32268=DIRECTION('center_axis',(0.,-1.,0.));
#32269=DIRECTION('ref_axis',(0.,0.,-1.));
#32270=DIRECTION('center_axis',(0.,1.,0.));
#32271=DIRECTION('ref_axis',(0.707106781186546,0.,-0.707106781186549));
#32272=DIRECTION('center_axis',(0.,-1.,0.));
#32273=DIRECTION('ref_axis',(0.,0.,-1.));
#32274=DIRECTION('center_axis',(-1.,0.,0.));
#32275=DIRECTION('ref_axis',(0.,0.,1.));
#32276=DIRECTION('center_axis',(1.,0.,0.));
#32277=DIRECTION('ref_axis',(0.,-1.,-1.48029736616687E-15));
#32278=DIRECTION('',(1.,0.,0.));
#32279=DIRECTION('',(1.,0.,0.));
#32280=DIRECTION('center_axis',(0.,0.,-1.));
#32281=DIRECTION('ref_axis',(0.,1.,0.));
#32282=DIRECTION('',(1.,0.,0.));
#32283=DIRECTION('center_axis',(1.,0.,0.));
#32284=DIRECTION('ref_axis',(0.,0.,-1.));
#32285=DIRECTION('center_axis',(0.,1.,0.));
#32286=DIRECTION('ref_axis',(1.,0.,0.));
#32287=DIRECTION('center_axis',(0.,1.,0.));
#32288=DIRECTION('ref_axis',(1.,0.,0.));
#32289=DIRECTION('center_axis',(0.,1.,0.));
#32290=DIRECTION('ref_axis',(1.,0.,0.));
#32291=DIRECTION('center_axis',(0.,1.,0.));
#32292=DIRECTION('ref_axis',(1.,0.,0.));
#32293=DIRECTION('center_axis',(0.,-1.,0.));
#32294=DIRECTION('ref_axis',(1.,0.,0.));
#32295=DIRECTION('',(0.,-1.,0.));
#32296=DIRECTION('center_axis',(0.,-1.,0.));
#32297=DIRECTION('ref_axis',(1.,0.,0.));
#32298=DIRECTION('',(0.,-1.,0.));
#32299=DIRECTION('center_axis',(0.,-1.,0.));
#32300=DIRECTION('ref_axis',(1.,0.,0.));
#32301=DIRECTION('',(0.,-1.,0.));
#32302=DIRECTION('center_axis',(0.,-1.,0.));
#32303=DIRECTION('ref_axis',(1.,0.,0.));
#32304=DIRECTION('',(0.,-1.,0.));
#32305=DIRECTION('center_axis',(0.,-1.,0.));
#32306=DIRECTION('ref_axis',(0.,0.,-1.));
#32307=DIRECTION('center_axis',(0.,0.,-1.));
#32308=DIRECTION('ref_axis',(0.,-1.,0.));
#32309=DIRECTION('center_axis',(0.,-1.,0.));
#32310=DIRECTION('ref_axis',(0.,0.,-1.));
#32311=DIRECTION('center_axis',(0.,1.,0.));
#32312=DIRECTION('ref_axis',(1.,0.,0.));
#32313=DIRECTION('center_axis',(0.,1.,0.));
#32314=DIRECTION('ref_axis',(0.,0.,1.));
#32315=DIRECTION('center_axis',(0.,1.,0.));
#32316=DIRECTION('ref_axis',(0.,0.,1.));
#32317=DIRECTION('',(0.,1.,0.));
#32318=DIRECTION('center_axis',(0.,-1.,0.));
#32319=DIRECTION('ref_axis',(0.,0.,-1.));
#32320=DIRECTION('center_axis',(0.,1.,0.));
#32321=DIRECTION('ref_axis',(1.,0.,0.));
#32322=DIRECTION('center_axis',(0.,1.,0.));
#32323=DIRECTION('ref_axis',(0.,0.,1.));
#32324=DIRECTION('center_axis',(0.,1.,0.));
#32325=DIRECTION('ref_axis',(0.,0.,1.));
#32326=DIRECTION('',(0.,1.,0.));
#32327=DIRECTION('center_axis',(0.,1.,0.));
#32328=DIRECTION('ref_axis',(2.96059473233374E-15,0.,1.));
#32329=DIRECTION('',(0.,1.,0.));
#32330=DIRECTION('center_axis',(0.,0.,1.));
#32331=DIRECTION('ref_axis',(1.,0.,0.));
#32332=DIRECTION('',(0.,1.,0.));
#32333=DIRECTION('center_axis',(0.,1.,0.));
#32334=DIRECTION('ref_axis',(-1.,0.,2.96059473233374E-15));
#32335=DIRECTION('center_axis',(0.,0.,-1.));
#32336=DIRECTION('ref_axis',(-1.,0.,0.));
#32337=DIRECTION('',(0.,1.,0.));
#32338=DIRECTION('center_axis',(0.,1.,0.));
#32339=DIRECTION('ref_axis',(1.,0.,-2.96059473233374E-15));
#32340=DIRECTION('center_axis',(1.,0.,0.));
#32341=DIRECTION('ref_axis',(0.,1.,0.));
#32342=DIRECTION('',(0.,0.,1.));
#32343=DIRECTION('center_axis',(0.,0.,1.));
#32344=DIRECTION('ref_axis',(0.,-1.,0.));
#32345=DIRECTION('',(0.,0.,1.));
#32346=DIRECTION('center_axis',(0.,-1.,0.));
#32347=DIRECTION('ref_axis',(1.,0.,0.));
#32348=DIRECTION('',(0.,0.,1.));
#32349=DIRECTION('center_axis',(0.,0.,1.));
#32350=DIRECTION('ref_axis',(-1.,0.,0.));
#32351=DIRECTION('center_axis',(0.,-1.,0.));
#32352=DIRECTION('ref_axis',(1.,0.,0.));
#32353=DIRECTION('',(0.,0.,1.));
#32354=DIRECTION('',(0.,0.,1.));
#32355=DIRECTION('center_axis',(0.,0.,1.));
#32356=DIRECTION('ref_axis',(-1.,0.,0.));
#32357=DIRECTION('',(0.,0.,1.));
#32358=DIRECTION('center_axis',(-1.,0.,0.));
#32359=DIRECTION('ref_axis',(0.,-1.,0.));
#32360=DIRECTION('',(0.,0.,1.));
#32361=DIRECTION('center_axis',(0.,0.,1.));
#32362=DIRECTION('ref_axis',(4.44089209850064E-15,1.,0.));
#32363=DIRECTION('',(0.,0.,1.));
#32364=DIRECTION('center_axis',(0.,1.,0.));
#32365=DIRECTION('ref_axis',(-1.,0.,0.));
#32366=DIRECTION('',(0.,0.,1.));
#32367=DIRECTION('center_axis',(0.,0.,1.));
#32368=DIRECTION('ref_axis',(1.,0.,0.));
#32369=DIRECTION('',(0.,0.,1.));
#32370=DIRECTION('center_axis',(1.,0.,0.));
#32371=DIRECTION('ref_axis',(0.,1.,0.));
#32372=DIRECTION('',(0.,0.,1.));
#32373=DIRECTION('center_axis',(0.,0.,1.));
#32374=DIRECTION('ref_axis',(-4.44089209850064E-15,-1.,0.));
#32375=DIRECTION('center_axis',(0.,0.,1.));
#32376=DIRECTION('ref_axis',(1.,0.,0.));
#32377=DIRECTION('',(0.,1.,0.));
#32378=DIRECTION('',(0.,1.,0.));
#32379=DIRECTION('center_axis',(0.,1.,0.));
#32380=DIRECTION('ref_axis',(-1.,0.,0.));
#32381=DIRECTION('center_axis',(0.,1.,0.));
#32382=DIRECTION('ref_axis',(0.,0.,1.));
#32383=DIRECTION('center_axis',(0.,1.,0.));
#32384=DIRECTION('ref_axis',(0.,0.,1.));
#32385=DIRECTION('',(0.,-1.,0.));
#32386=DIRECTION('center_axis',(0.,-1.,0.));
#32387=DIRECTION('ref_axis',(0.,0.,1.));
#32388=DIRECTION('',(-8.48405894740086E-18,-0.99759742096768,-0.0692775986783111));
#41492=CARTESIAN_POINT('',(0.,0.,0.));
#41493=CARTESIAN_POINT('Origin',(0.,133.75,0.));
#41494=CARTESIAN_POINT('',(-3.24653866453963E-15,134.,-26.51));
#41495=CARTESIAN_POINT('Origin',(0.,134.,0.));
#41496=CARTESIAN_POINT('',(3.18530632458227E-15,133.5,-26.01));
#41497=CARTESIAN_POINT('',(-3.21592249456095E-15,133.75,-26.26));
#41498=CARTESIAN_POINT('Origin',(0.,133.5,0.));
#41499=CARTESIAN_POINT('Origin',(0.,100.05,0.));
#41500=CARTESIAN_POINT('',(-3.18530632458227E-15,130.65,-26.01));
#41501=CARTESIAN_POINT('Origin',(0.,130.65,0.));
#41502=CARTESIAN_POINT('',(-3.18530632458227E-15,100.05,-26.01));
#41503=CARTESIAN_POINT('Origin',(0.,134.,0.));
#41504=CARTESIAN_POINT('',(47.,134.,-41.));
#41505=CARTESIAN_POINT('',(41.,134.,-47.));
#41506=CARTESIAN_POINT('Origin',(41.,134.,-41.));
#41507=CARTESIAN_POINT('',(-41.,134.,-47.));
#41508=CARTESIAN_POINT('',(-41.,134.,-47.));
#41509=CARTESIAN_POINT('',(-47.,134.,-41.));
#41510=CARTESIAN_POINT('Origin',(-41.,134.,-41.));
#41511=CARTESIAN_POINT('',(-47.,134.,41.));
#41512=CARTESIAN_POINT('',(-47.,134.,41.));
#41513=CARTESIAN_POINT('',(-41.,134.,47.));
#41514=CARTESIAN_POINT('Origin',(-41.,134.,41.));
#41515=CARTESIAN_POINT('',(41.,134.,47.));
#41516=CARTESIAN_POINT('',(41.,134.,47.));
#41517=CARTESIAN_POINT('',(47.,134.,41.));
#41518=CARTESIAN_POINT('Origin',(41.,134.,41.));
#41519=CARTESIAN_POINT('',(47.,134.,-41.));
#41520=CARTESIAN_POINT('Origin',(0.,130.4,0.));
#41521=CARTESIAN_POINT('',(3.24653866453963E-15,130.15,-26.51));
#41522=CARTESIAN_POINT('',(-3.21592249456095E-15,130.4,-26.26));
#41523=CARTESIAN_POINT('Origin',(0.,130.15,0.));
#41524=CARTESIAN_POINT('Origin',(0.,130.15,25.9));
#41525=CARTESIAN_POINT('',(-3.36777869765522E-15,130.15,-27.5));
#41526=CARTESIAN_POINT('Origin',(0.,130.15,0.));
#41527=CARTESIAN_POINT('Origin',(60.,190.,-125.25));
#41528=CARTESIAN_POINT('',(52.5,190.,-125.));
#41529=CARTESIAN_POINT('Origin',(60.,190.,-125.));
#41530=CARTESIAN_POINT('',(53.,190.,-125.5));
#41531=CARTESIAN_POINT('',(52.75,190.,-125.25));
#41532=CARTESIAN_POINT('Origin',(60.,190.,-125.5));
#41533=CARTESIAN_POINT('Origin',(0.,182.5,-125.));
#41534=CARTESIAN_POINT('',(-75.,164.,-125.));
#41535=CARTESIAN_POINT('',(-71.,160.,-125.));
#41536=CARTESIAN_POINT('Origin',(-71.,164.,-125.));
#41537=CARTESIAN_POINT('',(71.,160.,-125.));
#41538=CARTESIAN_POINT('',(-71.,160.,-125.));
#41539=CARTESIAN_POINT('',(75.,164.,-125.));
#41540=CARTESIAN_POINT('Origin',(71.,164.,-125.));
#41541=CARTESIAN_POINT('',(75.,201.,-125.));
#41542=CARTESIAN_POINT('',(75.,164.,-125.));
#41543=CARTESIAN_POINT('',(71.,205.,-125.));
#41544=CARTESIAN_POINT('Origin',(71.,201.,-125.));
#41545=CARTESIAN_POINT('',(0.,205.,-125.));
#41546=CARTESIAN_POINT('',(71.,205.,-125.));
#41547=CARTESIAN_POINT('',(0.,204.5,-125.));
#41548=CARTESIAN_POINT('',(0.,209.75,-125.));
#41549=CARTESIAN_POINT('',(-71.,205.,-125.));
#41550=CARTESIAN_POINT('',(71.,205.,-125.));
#41551=CARTESIAN_POINT('',(-75.,201.,-125.));
#41552=CARTESIAN_POINT('Origin',(-71.,201.,-125.));
#41553=CARTESIAN_POINT('',(-75.,201.,-125.));
#41554=CARTESIAN_POINT('',(-67.5,190.,-125.));
#41555=CARTESIAN_POINT('Origin',(-60.,190.,-125.));
#41556=CARTESIAN_POINT('',(-36.,165.,-125.));
#41557=CARTESIAN_POINT('',(36.,165.,-125.));
#41558=CARTESIAN_POINT('',(-36.,165.,-125.));
#41559=CARTESIAN_POINT('',(-40.,169.,-125.));
#41560=CARTESIAN_POINT('Origin',(-36.,169.,-125.));
#41561=CARTESIAN_POINT('',(-40.,196.,-125.));
#41562=CARTESIAN_POINT('',(-40.,196.,-125.));
#41563=CARTESIAN_POINT('',(-36.,200.,-125.));
#41564=CARTESIAN_POINT('Origin',(-36.,196.,-125.));
#41565=CARTESIAN_POINT('',(36.,200.,-125.));
#41566=CARTESIAN_POINT('',(36.,200.,-125.));
#41567=CARTESIAN_POINT('',(40.,196.,-125.));
#41568=CARTESIAN_POINT('Origin',(36.,196.,-125.));
#41569=CARTESIAN_POINT('',(40.,169.,-125.));
#41570=CARTESIAN_POINT('',(40.,169.,-125.));
#41571=CARTESIAN_POINT('Origin',(36.,169.,-125.));
#41572=CARTESIAN_POINT('Origin',(60.,190.,-125.));
#41573=CARTESIAN_POINT('',(53.,190.,-139.5));
#41574=CARTESIAN_POINT('',(53.,190.,-125.));
#41575=CARTESIAN_POINT('Origin',(60.,190.,-139.5));
#41576=CARTESIAN_POINT('Origin',(-60.,190.,-125.25));
#41577=CARTESIAN_POINT('',(-67.,190.,-125.5));
#41578=CARTESIAN_POINT('',(-67.25,190.,-125.25));
#41579=CARTESIAN_POINT('Origin',(-60.,190.,-125.5));
#41580=CARTESIAN_POINT('Origin',(-60.,190.,-125.));
#41581=CARTESIAN_POINT('',(-67.,190.,-139.5));
#41582=CARTESIAN_POINT('',(-67.,190.,-125.));
#41583=CARTESIAN_POINT('Origin',(-60.,190.,-139.5));
#41584=CARTESIAN_POINT('Origin',(-47.25,193.,38.));
#41585=CARTESIAN_POINT('',(-47.,193.55,41.));
#41586=CARTESIAN_POINT('',(-47.5,193.459836065574,40.5081967213115));
#41587=CARTESIAN_POINT('',(-47.,193.55,41.));
#41588=CARTESIAN_POINT('',(-47.5,192.540163934426,40.5081967213115));
#41589=CARTESIAN_POINT('Origin',(-47.5,193.,38.));
#41590=CARTESIAN_POINT('',(-47.,192.45,41.));
#41591=CARTESIAN_POINT('',(-47.5,192.540163934426,40.5081967213115));
#41592=CARTESIAN_POINT('Origin',(-47.,193.,38.));
#41593=CARTESIAN_POINT('Ctrl Pts',(-47.,192.45,41.));
#41594=CARTESIAN_POINT('Ctrl Pts',(-47.,192.812639548803,41.0664839172805));
#41595=CARTESIAN_POINT('Ctrl Pts',(-47.,193.187360451197,41.0664839172805));
#41596=CARTESIAN_POINT('Ctrl Pts',(-47.,193.55,41.));
#41597=CARTESIAN_POINT('Ctrl Pts',(-47.1666666666667,192.480054644809,40.8360655737705));
#41598=CARTESIAN_POINT('Ctrl Pts',(-47.1666666666667,192.822877824825,40.8989164901067));
#41599=CARTESIAN_POINT('Ctrl Pts',(-47.1666666666667,193.177122175175,40.8989164901067));
#41600=CARTESIAN_POINT('Ctrl Pts',(-47.1666666666667,193.519945355191,40.8360655737705));
#41601=CARTESIAN_POINT('Ctrl Pts',(-47.3333333333333,192.510109289617,40.672131147541));
#41602=CARTESIAN_POINT('Ctrl Pts',(-47.3333333333333,192.833116100846,40.7313490629329));
#41603=CARTESIAN_POINT('Ctrl Pts',(-47.3333333333333,193.166883899154,40.7313490629329));
#41604=CARTESIAN_POINT('Ctrl Pts',(-47.3333333333333,193.489890710383,40.672131147541));
#41605=CARTESIAN_POINT('Ctrl Pts',(-47.5,192.540163934426,40.5081967213115));
#41606=CARTESIAN_POINT('Ctrl Pts',(-47.5,192.843354376868,40.5637816357591));
#41607=CARTESIAN_POINT('Ctrl Pts',(-47.5,193.156645623132,40.5637816357591));
#41608=CARTESIAN_POINT('Ctrl Pts',(-47.5,193.459836065574,40.5081967213115));
#41609=CARTESIAN_POINT('Ctrl Pts',(-47.,193.55,41.));
#41610=CARTESIAN_POINT('Ctrl Pts',(-47.,193.187360451197,41.0664839172805));
#41611=CARTESIAN_POINT('Ctrl Pts',(-47.,192.812639548803,41.0664839172805));
#41612=CARTESIAN_POINT('Ctrl Pts',(-47.,192.45,41.));
#41613=CARTESIAN_POINT('',(-47.5,193.,40.5498854071472));
#41614=CARTESIAN_POINT('Ctrl Pts',(-47.5,192.540163934426,40.5081967213115));
#41615=CARTESIAN_POINT('Ctrl Pts',(-47.5,192.691759155647,40.5359891785353));
#41616=CARTESIAN_POINT('Ctrl Pts',(-47.5,192.845879577824,40.5498854071472));
#41617=CARTESIAN_POINT('Ctrl Pts',(-47.5,193.,40.5498854071472));
#41618=CARTESIAN_POINT('Ctrl Pts',(-47.5,193.,40.5498854071472));
#41619=CARTESIAN_POINT('Ctrl Pts',(-47.5,193.154120422176,40.5498854071472));
#41620=CARTESIAN_POINT('Ctrl Pts',(-47.5,193.308240844353,40.5359891785353));
#41621=CARTESIAN_POINT('Ctrl Pts',(-47.5,193.459836065574,40.5081967213115));
#41622=CARTESIAN_POINT('Origin',(-47.,134.,-41.));
#41623=CARTESIAN_POINT('',(-47.,141.55,41.));
#41624=CARTESIAN_POINT('',(-47.,134.,41.));
#41625=CARTESIAN_POINT('',(-47.,140.45,41.));
#41626=CARTESIAN_POINT('Origin',(-47.,141.,38.));
#41627=CARTESIAN_POINT('',(-47.,134.,41.));
#41628=CARTESIAN_POINT('',(-47.,140.45,-41.));
#41629=CARTESIAN_POINT('',(-47.,134.,-41.));
#41630=CARTESIAN_POINT('',(-47.,141.55,-41.));
#41631=CARTESIAN_POINT('Origin',(-47.,141.,-38.));
#41632=CARTESIAN_POINT('',(-47.,192.45,-41.));
#41633=CARTESIAN_POINT('',(-47.,134.,-41.));
#41634=CARTESIAN_POINT('',(-47.,193.55,-41.));
#41635=CARTESIAN_POINT('Origin',(-47.,193.,-38.));
#41636=CARTESIAN_POINT('',(-47.,203.,-41.));
#41637=CARTESIAN_POINT('',(-47.,134.,-41.));
#41638=CARTESIAN_POINT('',(-47.,203.,0.));
#41639=CARTESIAN_POINT('',(-47.,203.,41.));
#41640=CARTESIAN_POINT('',(-47.,203.,41.));
#41641=CARTESIAN_POINT('',(-47.,203.,41.));
#41642=CARTESIAN_POINT('',(-47.,134.,41.));
#41643=CARTESIAN_POINT('',(-47.,194.,-24.));
#41644=CARTESIAN_POINT('',(-47.,194.,24.));
#41645=CARTESIAN_POINT('',(-47.,194.,-32.5));
#41646=CARTESIAN_POINT('',(-47.,186.,-32.));
#41647=CARTESIAN_POINT('Origin',(-47.,186.,-24.));
#41648=CARTESIAN_POINT('',(-47.,148.,-32.));
#41649=CARTESIAN_POINT('',(-47.,141.,-32.));
#41650=CARTESIAN_POINT('',(-47.,140.,-24.));
#41651=CARTESIAN_POINT('Origin',(-47.,148.,-24.));
#41652=CARTESIAN_POINT('',(-47.,140.,24.));
#41653=CARTESIAN_POINT('',(-47.,140.,-8.5));
#41654=CARTESIAN_POINT('',(-47.,148.,32.));
#41655=CARTESIAN_POINT('Origin',(-47.,148.,24.));
#41656=CARTESIAN_POINT('',(-47.,186.,32.));
#41657=CARTESIAN_POINT('',(-47.,160.,32.));
#41658=CARTESIAN_POINT('Origin',(-47.,186.,24.));
#41659=CARTESIAN_POINT('Origin',(-55.,193.,38.));
#41660=CARTESIAN_POINT('',(-54.5,193.,40.55));
#41661=CARTESIAN_POINT('Origin',(-54.5,193.,38.));
#41662=CARTESIAN_POINT('',(-55.,193.,40.55));
#41663=CARTESIAN_POINT('Origin',(-47.25,141.,-38.));
#41664=CARTESIAN_POINT('',(-47.5,140.540163934426,-40.5081967213115));
#41665=CARTESIAN_POINT('',(-47.,140.45,-41.));
#41666=CARTESIAN_POINT('',(-47.5,141.,-35.45));
#41667=CARTESIAN_POINT('Origin',(-47.5,141.,-38.));
#41668=CARTESIAN_POINT('',(-47.5,141.459836065574,-40.5081967213115));
#41669=CARTESIAN_POINT('Origin',(-47.5,141.,-38.));
#41670=CARTESIAN_POINT('',(-47.5,141.459836065574,-40.5081967213115));
#41671=CARTESIAN_POINT('Ctrl Pts',(-47.,141.55,-41.));
#41672=CARTESIAN_POINT('Ctrl Pts',(-47.,141.187360451197,-41.0664839172806));
#41673=CARTESIAN_POINT('Ctrl Pts',(-47.,140.812639548803,-41.0664839172805));
#41674=CARTESIAN_POINT('Ctrl Pts',(-47.,140.45,-41.));
#41675=CARTESIAN_POINT('Ctrl Pts',(-47.1666666666667,141.519945355191,-40.8360655737705));
#41676=CARTESIAN_POINT('Ctrl Pts',(-47.1666666666667,141.177122175175,-40.8989164901067));
#41677=CARTESIAN_POINT('Ctrl Pts',(-47.1666666666667,140.822877824825,-40.8989164901067));
#41678=CARTESIAN_POINT('Ctrl Pts',(-47.1666666666667,140.480054644809,-40.8360655737705));
#41679=CARTESIAN_POINT('Ctrl Pts',(-47.3333333333333,141.489890710382,-40.672131147541));
#41680=CARTESIAN_POINT('Ctrl Pts',(-47.3333333333333,141.166883899154,-40.7313490629329));
#41681=CARTESIAN_POINT('Ctrl Pts',(-47.3333333333333,140.833116100846,-40.7313490629329));
#41682=CARTESIAN_POINT('Ctrl Pts',(-47.3333333333333,140.510109289617,-40.672131147541));
#41683=CARTESIAN_POINT('Ctrl Pts',(-47.5,141.459836065574,-40.5081967213115));
#41684=CARTESIAN_POINT('Ctrl Pts',(-47.5,141.156645623132,-40.5637816357591));
#41685=CARTESIAN_POINT('Ctrl Pts',(-47.5,140.843354376868,-40.5637816357591));
#41686=CARTESIAN_POINT('Ctrl Pts',(-47.5,140.540163934426,-40.5081967213115));
#41687=CARTESIAN_POINT('Ctrl Pts',(-47.,140.45,-41.));
#41688=CARTESIAN_POINT('Ctrl Pts',(-47.,140.812639548803,-41.0664839172805));
#41689=CARTESIAN_POINT('Ctrl Pts',(-47.,141.187360451197,-41.0664839172806));
#41690=CARTESIAN_POINT('Ctrl Pts',(-47.,141.55,-41.));
#41691=CARTESIAN_POINT('Ctrl Pts',(-47.5,141.459836065574,-40.5081967213115));
#41692=CARTESIAN_POINT('Ctrl Pts',(-47.5,141.156645623132,-40.5637816357591));
#41693=CARTESIAN_POINT('Ctrl Pts',(-47.5,140.843354376868,-40.5637816357591));
#41694=CARTESIAN_POINT('Ctrl Pts',(-47.5,140.540163934426,-40.5081967213115));
#41695=CARTESIAN_POINT('Origin',(-41.,134.,-41.));
#41696=CARTESIAN_POINT('',(-41.,203.,-47.));
#41697=CARTESIAN_POINT('',(-41.,134.,-47.));
#41698=CARTESIAN_POINT('Origin',(-41.,203.,-41.));
#41699=CARTESIAN_POINT('Ctrl Pts',(-47.,192.45,-41.));
#41700=CARTESIAN_POINT('Ctrl Pts',(-47.,192.812639548803,-41.0664839172806));
#41701=CARTESIAN_POINT('Ctrl Pts',(-47.,193.187360451197,-41.0664839172806));
#41702=CARTESIAN_POINT('Ctrl Pts',(-47.,193.55,-41.));
#41703=CARTESIAN_POINT('Origin',(-55.,141.,-38.));
#41704=CARTESIAN_POINT('',(-54.5,141.,-35.45));
#41705=CARTESIAN_POINT('Origin',(-54.5,141.,-38.));
#41706=CARTESIAN_POINT('',(-55.,141.,-35.45));
#41707=CARTESIAN_POINT('Origin',(-47.25,141.,38.));
#41708=CARTESIAN_POINT('',(-47.5,141.459836065574,40.5081967213115));
#41709=CARTESIAN_POINT('',(-47.,141.55,41.));
#41710=CARTESIAN_POINT('',(-47.5,140.540163934426,40.5081967213115));
#41711=CARTESIAN_POINT('Origin',(-47.5,141.,38.));
#41712=CARTESIAN_POINT('',(-47.5,140.540163934426,40.5081967213115));
#41713=CARTESIAN_POINT('Ctrl Pts',(-47.,140.45,41.));
#41714=CARTESIAN_POINT('Ctrl Pts',(-47.,140.812639548803,41.0664839172806));
#41715=CARTESIAN_POINT('Ctrl Pts',(-47.,141.187360451197,41.0664839172805));
#41716=CARTESIAN_POINT('Ctrl Pts',(-47.,141.55,41.));
#41717=CARTESIAN_POINT('Ctrl Pts',(-47.1666666666667,140.480054644809,40.8360655737705));
#41718=CARTESIAN_POINT('Ctrl Pts',(-47.1666666666667,140.822877824825,40.8989164901067));
#41719=CARTESIAN_POINT('Ctrl Pts',(-47.1666666666667,141.177122175175,40.8989164901067));
#41720=CARTESIAN_POINT('Ctrl Pts',(-47.1666666666667,141.519945355191,40.8360655737705));
#41721=CARTESIAN_POINT('Ctrl Pts',(-47.3333333333333,140.510109289617,40.672131147541));
#41722=CARTESIAN_POINT('Ctrl Pts',(-47.3333333333333,140.833116100846,40.7313490629329));
#41723=CARTESIAN_POINT('Ctrl Pts',(-47.3333333333333,141.166883899154,40.7313490629329));
#41724=CARTESIAN_POINT('Ctrl Pts',(-47.3333333333333,141.489890710383,40.672131147541));
#41725=CARTESIAN_POINT('Ctrl Pts',(-47.5,140.540163934426,40.5081967213115));
#41726=CARTESIAN_POINT('Ctrl Pts',(-47.5,140.843354376868,40.5637816357591));
#41727=CARTESIAN_POINT('Ctrl Pts',(-47.5,141.156645623132,40.5637816357591));
#41728=CARTESIAN_POINT('Ctrl Pts',(-47.5,141.459836065574,40.5081967213115));
#41729=CARTESIAN_POINT('Ctrl Pts',(-47.,141.55,41.));
#41730=CARTESIAN_POINT('Ctrl Pts',(-47.,141.187360451197,41.0664839172805));
#41731=CARTESIAN_POINT('Ctrl Pts',(-47.,140.812639548803,41.0664839172806));
#41732=CARTESIAN_POINT('Ctrl Pts',(-47.,140.45,41.));
#41733=CARTESIAN_POINT('',(-47.5,141.,40.5498854071472));
#41734=CARTESIAN_POINT('Ctrl Pts',(-47.5,140.540163934426,40.5081967213115));
#41735=CARTESIAN_POINT('Ctrl Pts',(-47.5,140.691759155647,40.5359891785353));
#41736=CARTESIAN_POINT('Ctrl Pts',(-47.5,140.845879577824,40.5498854071472));
#41737=CARTESIAN_POINT('Ctrl Pts',(-47.5,141.,40.5498854071472));
#41738=CARTESIAN_POINT('Ctrl Pts',(-47.5,141.,40.5498854071472));
#41739=CARTESIAN_POINT('Ctrl Pts',(-47.5,141.154120422176,40.5498854071472));
#41740=CARTESIAN_POINT('Ctrl Pts',(-47.5,141.308240844353,40.5359891785353));
#41741=CARTESIAN_POINT('Ctrl Pts',(-47.5,141.459836065574,40.5081967213115));
#41742=CARTESIAN_POINT('Origin',(-55.,141.,38.));
#41743=CARTESIAN_POINT('',(-54.5,141.,40.55));
#41744=CARTESIAN_POINT('Origin',(-54.5,141.,38.));
#41745=CARTESIAN_POINT('',(-55.,141.,40.55));
#41746=CARTESIAN_POINT('Origin',(-47.25,193.,-38.));
#41747=CARTESIAN_POINT('',(-47.5,192.540163934426,-40.5081967213115));
#41748=CARTESIAN_POINT('',(-47.,192.45,-41.));
#41749=CARTESIAN_POINT('',(-47.5,193.,-35.45));
#41750=CARTESIAN_POINT('Origin',(-47.5,193.,-38.));
#41751=CARTESIAN_POINT('',(-47.5,193.459836065574,-40.5081967213115));
#41752=CARTESIAN_POINT('Origin',(-47.5,193.,-38.));
#41753=CARTESIAN_POINT('',(-47.5,193.459836065574,-40.5081967213115));
#41754=CARTESIAN_POINT('Ctrl Pts',(-47.,193.55,-41.));
#41755=CARTESIAN_POINT('Ctrl Pts',(-47.,193.187360451197,-41.0664839172806));
#41756=CARTESIAN_POINT('Ctrl Pts',(-47.,192.812639548803,-41.0664839172806));
#41757=CARTESIAN_POINT('Ctrl Pts',(-47.,192.45,-41.));
#41758=CARTESIAN_POINT('Ctrl Pts',(-47.1666666666667,193.519945355191,-40.8360655737705));
#41759=CARTESIAN_POINT('Ctrl Pts',(-47.1666666666667,193.177122175175,-40.8989164901067));
#41760=CARTESIAN_POINT('Ctrl Pts',(-47.1666666666667,192.822877824825,-40.8989164901067));
#41761=CARTESIAN_POINT('Ctrl Pts',(-47.1666666666667,192.480054644809,-40.8360655737705));
#41762=CARTESIAN_POINT('Ctrl Pts',(-47.3333333333333,193.489890710383,-40.672131147541));
#41763=CARTESIAN_POINT('Ctrl Pts',(-47.3333333333333,193.166883899154,-40.7313490629329));
#41764=CARTESIAN_POINT('Ctrl Pts',(-47.3333333333333,192.833116100846,-40.7313490629329));
#41765=CARTESIAN_POINT('Ctrl Pts',(-47.3333333333333,192.510109289617,-40.672131147541));
#41766=CARTESIAN_POINT('Ctrl Pts',(-47.5,193.459836065574,-40.5081967213115));
#41767=CARTESIAN_POINT('Ctrl Pts',(-47.5,193.156645623132,-40.5637816357591));
#41768=CARTESIAN_POINT('Ctrl Pts',(-47.5,192.843354376868,-40.5637816357591));
#41769=CARTESIAN_POINT('Ctrl Pts',(-47.5,192.540163934426,-40.5081967213115));
#41770=CARTESIAN_POINT('Ctrl Pts',(-47.5,193.459836065574,-40.5081967213115));
#41771=CARTESIAN_POINT('Ctrl Pts',(-47.5,193.156645623132,-40.5637816357591));
#41772=CARTESIAN_POINT('Ctrl Pts',(-47.5,192.843354376868,-40.5637816357591));
#41773=CARTESIAN_POINT('Ctrl Pts',(-47.5,192.540163934426,-40.5081967213115));
#41774=CARTESIAN_POINT('Origin',(-55.,193.,-38.));
#41775=CARTESIAN_POINT('',(-54.5,193.,-35.45));
#41776=CARTESIAN_POINT('Origin',(-54.5,193.,-38.));
#41777=CARTESIAN_POINT('',(-55.,193.,-35.45));
#41778=CARTESIAN_POINT('Origin',(-54.75,193.,-38.));
#41779=CARTESIAN_POINT('',(-55.,193.,-34.95));
#41780=CARTESIAN_POINT('Origin',(-55.,193.,-38.));
#41781=CARTESIAN_POINT('',(-54.75,193.,-35.2));
#41782=CARTESIAN_POINT('Origin',(-55.,130.,-47.));
#41783=CARTESIAN_POINT('',(-55.,132.,47.));
#41784=CARTESIAN_POINT('',(-55.,132.,-47.));
#41785=CARTESIAN_POINT('',(-55.,132.,-23.5));
#41786=CARTESIAN_POINT('',(-55.,199.531133844866,47.));
#41787=CARTESIAN_POINT('',(-55.,130.,47.));
#41788=CARTESIAN_POINT('',(-55.,199.004037328772,32.85003536606));
#41789=CARTESIAN_POINT('Ctrl Pts',(-55.,199.531133844866,47.0000000000002));
#41790=CARTESIAN_POINT('Ctrl Pts',(-55.,199.22088305859,39.4954174846766));
#41791=CARTESIAN_POINT('Ctrl Pts',(-55.,199.004037328771,32.8500353660488));
#41792=CARTESIAN_POINT('',(-55.,199.,32.6016382508379));
#41793=CARTESIAN_POINT('Ctrl Pts',(-55.,199.004037328772,32.85003536606));
#41794=CARTESIAN_POINT('Ctrl Pts',(-55.,199.001278753317,32.7654969801016));
#41795=CARTESIAN_POINT('Ctrl Pts',(-55.,199.,32.6824692460632));
#41796=CARTESIAN_POINT('Ctrl Pts',(-55.,199.,32.6016382508379));
#41797=CARTESIAN_POINT('',(-55.,199.,-32.6016382508379));
#41798=CARTESIAN_POINT('',(-55.,199.,8.5));
#41799=CARTESIAN_POINT('',(-55.,199.004037328772,-32.85003536606));
#41800=CARTESIAN_POINT('Ctrl Pts',(-55.,199.,-32.6016382508379));
#41801=CARTESIAN_POINT('Ctrl Pts',(-55.,199.,-32.6824692460632));
#41802=CARTESIAN_POINT('Ctrl Pts',(-55.,199.001278753317,-32.7654969801016));
#41803=CARTESIAN_POINT('Ctrl Pts',(-55.,199.004037328772,-32.85003536606));
#41804=CARTESIAN_POINT('',(-55.,199.531133844866,-47.));
#41805=CARTESIAN_POINT('Ctrl Pts',(-55.,199.004037328772,-32.85003536606));
#41806=CARTESIAN_POINT('Ctrl Pts',(-55.,199.22088305859,-39.4954174846828));
#41807=CARTESIAN_POINT('Ctrl Pts',(-55.,199.531133844866,-47.0000000000002));
#41808=CARTESIAN_POINT('',(-55.,130.,-47.));
#41809=CARTESIAN_POINT('',(-55.,141.,41.05));
#41810=CARTESIAN_POINT('Origin',(-55.,141.,38.));
#41811=CARTESIAN_POINT('',(-55.,193.,41.05));
#41812=CARTESIAN_POINT('Origin',(-55.,193.,38.));
#41813=CARTESIAN_POINT('',(-55.,194.,24.));
#41814=CARTESIAN_POINT('',(-55.,194.,-24.));
#41815=CARTESIAN_POINT('',(-55.,194.,-35.5));
#41816=CARTESIAN_POINT('',(-55.,186.,32.));
#41817=CARTESIAN_POINT('Origin',(-55.,186.,24.));
#41818=CARTESIAN_POINT('',(-55.,148.,32.));
#41819=CARTESIAN_POINT('',(-55.,158.,32.));
#41820=CARTESIAN_POINT('',(-55.,140.,24.));
#41821=CARTESIAN_POINT('Origin',(-55.,148.,24.));
#41822=CARTESIAN_POINT('',(-55.,140.,-24.));
#41823=CARTESIAN_POINT('',(-55.,140.,-11.5));
#41824=CARTESIAN_POINT('',(-55.,148.,-32.));
#41825=CARTESIAN_POINT('Origin',(-55.,148.,-24.));
#41826=CARTESIAN_POINT('',(-55.,186.,-32.));
#41827=CARTESIAN_POINT('',(-55.,139.,-32.));
#41828=CARTESIAN_POINT('Origin',(-55.,186.,-24.));
#41829=CARTESIAN_POINT('',(-55.,141.,-34.95));
#41830=CARTESIAN_POINT('Origin',(-55.,141.,-38.));
#41831=CARTESIAN_POINT('Origin',(-54.75,141.,38.));
#41832=CARTESIAN_POINT('',(-54.75,141.,40.8));
#41833=CARTESIAN_POINT('Origin',(-54.75,141.,-38.));
#41834=CARTESIAN_POINT('',(-54.75,141.,-35.2));
#41835=CARTESIAN_POINT('Origin',(-54.75,193.,38.));
#41836=CARTESIAN_POINT('',(-54.75,193.,40.8));
#41837=CARTESIAN_POINT('Origin',(-76.0139789775539,214.75,-76.0139789775538));
#41838=CARTESIAN_POINT('',(-83.5139789775539,215.,-76.0139789775538));
#41839=CARTESIAN_POINT('Origin',(-76.0139789775539,215.,-76.0139789775538));
#41840=CARTESIAN_POINT('',(-83.0139789775539,214.5,-76.0139789775538));
#41841=CARTESIAN_POINT('',(-83.2639789775539,214.75,-76.0139789775538));
#41842=CARTESIAN_POINT('Origin',(-76.0139789775539,214.5,-76.0139789775538));
#41843=CARTESIAN_POINT('Origin',(0.,215.,45.));
#41844=CARTESIAN_POINT('',(-1.50631556295124E-14,215.,-123.));
#41845=CARTESIAN_POINT('Origin',(0.,215.,0.));
#41846=CARTESIAN_POINT('',(-83.5139789775538,215.,76.0139789775539));
#41847=CARTESIAN_POINT('Origin',(-76.0139789775538,215.,76.0139789775539));
#41848=CARTESIAN_POINT('',(68.5139789775538,215.,-76.0139789775539));
#41849=CARTESIAN_POINT('Origin',(76.0139789775538,215.,-76.0139789775539));
#41850=CARTESIAN_POINT('',(-1.12789970201471E-14,215.,92.1));
#41851=CARTESIAN_POINT('Origin',(0.,215.,0.));
#41852=CARTESIAN_POINT('',(68.5139789775538,215.,76.0139789775539));
#41853=CARTESIAN_POINT('Origin',(76.0139789775539,215.,76.0139789775539));
#41854=CARTESIAN_POINT('Origin',(-76.0139789775539,202.9,-76.0139789775538));
#41855=CARTESIAN_POINT('',(-83.0139789775539,202.9,-76.0139789775538));
#41856=CARTESIAN_POINT('Origin',(-76.0139789775539,202.9,-76.0139789775538));
#41857=CARTESIAN_POINT('',(-83.0139789775539,202.9,-76.0139789775538));
#41858=CARTESIAN_POINT('Origin',(-76.0139789775538,214.75,76.0139789775539));
#41859=CARTESIAN_POINT('',(-83.0139789775539,214.5,76.0139789775539));
#41860=CARTESIAN_POINT('',(-83.2639789775538,214.75,76.0139789775539));
#41861=CARTESIAN_POINT('Origin',(-76.0139789775538,214.5,76.0139789775539));
#41862=CARTESIAN_POINT('Origin',(-76.0139789775538,202.9,76.0139789775539));
#41863=CARTESIAN_POINT('',(-83.0139789775539,202.9,76.0139789775539));
#41864=CARTESIAN_POINT('Origin',(-76.0139789775538,202.9,76.0139789775539));
#41865=CARTESIAN_POINT('',(-83.0139789775539,202.9,76.0139789775539));
#41866=CARTESIAN_POINT('Origin',(76.0139789775539,214.75,76.0139789775539));
#41867=CARTESIAN_POINT('',(69.0139789775539,214.5,76.0139789775539));
#41868=CARTESIAN_POINT('',(68.7639789775538,214.75,76.0139789775539));
#41869=CARTESIAN_POINT('Origin',(76.0139789775539,214.5,76.0139789775539));
#41870=CARTESIAN_POINT('Origin',(76.0139789775539,202.9,76.0139789775539));
#41871=CARTESIAN_POINT('',(69.0139789775539,202.9,76.0139789775539));
#41872=CARTESIAN_POINT('Origin',(76.0139789775539,202.9,76.0139789775539));
#41873=CARTESIAN_POINT('',(69.0139789775539,202.9,76.0139789775539));
#41874=CARTESIAN_POINT('Origin',(76.0139789775538,214.75,-76.0139789775539));
#41875=CARTESIAN_POINT('',(69.0139789775538,214.5,-76.0139789775539));
#41876=CARTESIAN_POINT('',(68.7639789775538,214.75,-76.0139789775539));
#41877=CARTESIAN_POINT('Origin',(76.0139789775538,214.5,-76.0139789775539));
#41878=CARTESIAN_POINT('Origin',(76.0139789775538,202.9,-76.0139789775539));
#41879=CARTESIAN_POINT('',(69.0139789775538,202.9,-76.0139789775539));
#41880=CARTESIAN_POINT('Origin',(76.0139789775538,202.9,-76.0139789775539));
#41881=CARTESIAN_POINT('',(69.0139789775538,202.9,-76.0139789775539));
#41882=CARTESIAN_POINT('Origin',(-60.,190.,-139.75));
#41883=CARTESIAN_POINT('',(-67.5,190.,-140.));
#41884=CARTESIAN_POINT('Origin',(-60.,190.,-140.));
#41885=CARTESIAN_POINT('',(-67.25,190.,-139.75));
#41886=CARTESIAN_POINT('Origin',(0.,182.5,-140.));
#41887=CARTESIAN_POINT('',(-73.,201.,-140.));
#41888=CARTESIAN_POINT('',(-73.,164.,-140.));
#41889=CARTESIAN_POINT('',(-73.,191.75,-140.));
#41890=CARTESIAN_POINT('',(-71.,203.,-140.));
#41891=CARTESIAN_POINT('Origin',(-71.,201.,-140.));
#41892=CARTESIAN_POINT('',(71.,203.,-140.));
#41893=CARTESIAN_POINT('',(35.5,203.,-140.));
#41894=CARTESIAN_POINT('',(73.,201.,-140.));
#41895=CARTESIAN_POINT('Origin',(71.,201.,-140.));
#41896=CARTESIAN_POINT('',(73.,164.,-140.));
#41897=CARTESIAN_POINT('',(73.,173.25,-140.));
#41898=CARTESIAN_POINT('',(71.,162.,-140.));
#41899=CARTESIAN_POINT('Origin',(71.,164.,-140.));
#41900=CARTESIAN_POINT('',(-71.,162.,-140.));
#41901=CARTESIAN_POINT('',(-35.5,162.,-140.));
#41902=CARTESIAN_POINT('Origin',(-71.,164.,-140.));
#41903=CARTESIAN_POINT('',(52.5,190.,-140.));
#41904=CARTESIAN_POINT('Origin',(60.,190.,-140.));
#41905=CARTESIAN_POINT('Origin',(60.,190.,-139.75));
#41906=CARTESIAN_POINT('',(52.75,190.,-139.75));
#41907=CARTESIAN_POINT('Origin',(0.,60.,0.));
#41908=CARTESIAN_POINT('',(-8.57252759403147E-15,60.,-70.));
#41909=CARTESIAN_POINT('Origin',(0.,60.,0.));
#41910=CARTESIAN_POINT('',(8.327598234202E-15,62.,-68.));
#41911=CARTESIAN_POINT('Origin',(-8.327598234202E-15,60.,-68.));
#41912=CARTESIAN_POINT('Origin',(0.,62.,0.));
#41913=CARTESIAN_POINT('Origin',(0.,55.,0.));
#41914=CARTESIAN_POINT('',(0.,50.,-70.));
#41915=CARTESIAN_POINT('',(-8.57252759403147E-15,55.,-70.));
#41916=CARTESIAN_POINT('Origin',(0.,50.,0.));
#41917=CARTESIAN_POINT('Origin',(0.,62.,45.));
#41918=CARTESIAN_POINT('',(-46.5121933088198,62.,-41.0121933088198));
#41919=CARTESIAN_POINT('Origin',(-41.0121933088198,62.,-41.0121933088198));
#41920=CARTESIAN_POINT('',(-46.5121933088198,62.,41.0121933088198));
#41921=CARTESIAN_POINT('Origin',(-41.0121933088198,62.,41.0121933088198));
#41922=CARTESIAN_POINT('',(35.5121933088198,62.,41.0121933088198));
#41923=CARTESIAN_POINT('Origin',(41.0121933088198,62.,41.0121933088198));
#41924=CARTESIAN_POINT('',(35.5121933088197,62.,-41.0121933088198));
#41925=CARTESIAN_POINT('Origin',(41.0121933088197,62.,-41.0121933088198));
#41926=CARTESIAN_POINT('',(-5.51091059616309E-15,62.,-45.));
#41927=CARTESIAN_POINT('Origin',(0.,62.,0.));
#41928=CARTESIAN_POINT('Origin',(0.,50.,0.));
#41929=CARTESIAN_POINT('',(-1.6655196468404E-14,48.,-68.));
#41930=CARTESIAN_POINT('Origin',(0.,50.,-68.));
#41931=CARTESIAN_POINT('Origin',(0.,48.,0.));
#41932=CARTESIAN_POINT('Origin',(0.,48.,69.));
#41933=CARTESIAN_POINT('',(-2.75545529808154E-15,48.,-22.5));
#41934=CARTESIAN_POINT('Origin',(0.,48.,0.));
#41935=CARTESIAN_POINT('',(35.5121933088197,48.,-41.0121933088198));
#41936=CARTESIAN_POINT('Origin',(41.0121933088197,48.,-41.0121933088198));
#41937=CARTESIAN_POINT('',(35.5121933088198,48.,41.0121933088198));
#41938=CARTESIAN_POINT('Origin',(41.0121933088198,48.,41.0121933088198));
#41939=CARTESIAN_POINT('',(-46.5121933088198,48.,41.0121933088198));
#41940=CARTESIAN_POINT('Origin',(-41.0121933088198,48.,41.0121933088198));
#41941=CARTESIAN_POINT('',(-46.5121933088198,48.,-41.0121933088198));
#41942=CARTESIAN_POINT('Origin',(-41.0121933088198,48.,-41.0121933088198));
#41943=CARTESIAN_POINT('Origin',(0.,205.34240297561,0.));
#41944=CARTESIAN_POINT('',(-1.52380583888621E-14,203.928189413237,-124.428189413237));
#41945=CARTESIAN_POINT('Origin',(-1.14285437916466E-14,203.928189413237,
0.));
#41946=CARTESIAN_POINT('',(-1.51129017770466E-14,203.381241624228,-123.40620812114));
#41947=CARTESIAN_POINT('Origin',(-1.5064867177615E-14,205.34240297561,-123.013975850864));
#41948=CARTESIAN_POINT('Origin',(-1.1334676332785E-14,203.381241624228,
0.));
#41949=CARTESIAN_POINT('Origin',(0.,203.,0.));
#41950=CARTESIAN_POINT('',(-1.45893939117854E-14,202.526288399142,-119.131441995709));
#41951=CARTESIAN_POINT('',(-1.48794586096403E-14,203.,-121.5));
#41952=CARTESIAN_POINT('Origin',(-1.09420454338391E-14,202.526288399142,
0.));
#41953=CARTESIAN_POINT('Origin',(0.,204.,0.));
#41954=CARTESIAN_POINT('Origin',(0.,204.5,0.));
#41955=CARTESIAN_POINT('',(-1.52468526493845E-14,204.,-124.5));
#41956=CARTESIAN_POINT('Origin',(0.,204.487449750524,0.));
#41957=CARTESIAN_POINT('',(-1.45569142624227E-14,202.491487079295,-118.866225531784));
#41958=CARTESIAN_POINT('Origin',(-1.45413593123538E-14,204.487449750524,
-118.739209725433));
#41959=CARTESIAN_POINT('Origin',(-1.0917685696817E-14,202.491487079295,
0.));
#41960=CARTESIAN_POINT('Origin',(0.,200.75,0.));
#41961=CARTESIAN_POINT('',(-9.76218448463178E-15,200.,-79.7142857142859));
#41962=CARTESIAN_POINT('',(-1.12055182121983E-14,200.75,-91.5));
#41963=CARTESIAN_POINT('',(-36.,200.,-71.1222000991162));
#41964=CARTESIAN_POINT('Origin',(0.,200.,0.));
#41965=CARTESIAN_POINT('',(-38.4051782991124,199.196109721127,-55.));
#41966=CARTESIAN_POINT('Ctrl Pts',(-36.0000000000003,200.,-71.1222000991167));
#41967=CARTESIAN_POINT('Ctrl Pts',(-36.007998757625,200.,-71.1181513594252));
#41968=CARTESIAN_POINT('Ctrl Pts',(-36.0158673510785,199.999975166862,-71.1137294166545));
#41969=CARTESIAN_POINT('Ctrl Pts',(-36.0580820607069,199.999730794732,-71.088038844852));
#41970=CARTESIAN_POINT('Ctrl Pts',(-36.0894047422404,199.999088235995,-71.0608151548038));
#41971=CARTESIAN_POINT('Ctrl Pts',(-36.2557708347516,199.994267844983,-70.8912518979424));
#41972=CARTESIAN_POINT('Ctrl Pts',(-36.3559669090463,199.984858677538,-70.6735956916314));
#41973=CARTESIAN_POINT('Ctrl Pts',(-36.5729453400847,199.961300812392,-70.1447351250176));
#41974=CARTESIAN_POINT('Ctrl Pts',(-36.6773890334391,199.943421017973,-69.7728383598107));
#41975=CARTESIAN_POINT('Ctrl Pts',(-36.8678693651456,199.905921405603,-69.0049790361478));
#41976=CARTESIAN_POINT('Ctrl Pts',(-36.9507101031668,199.886166180182,-68.6082338248749));
#41977=CARTESIAN_POINT('Ctrl Pts',(-37.1771778906456,199.826039691768,-67.4102186809141));
#41978=CARTESIAN_POINT('Ctrl Pts',(-37.2985629364648,199.784876737986,-66.6023010705812));
#41979=CARTESIAN_POINT('Ctrl Pts',(-37.6420334379314,199.656620586686,-64.0895799742341));
#41980=CARTESIAN_POINT('Ctrl Pts',(-37.8330351423798,199.560609339382,-62.2193907504963));
#41981=CARTESIAN_POINT('Ctrl Pts',(-38.1547759803838,199.374640295943,-58.5623760439489));
#41982=CARTESIAN_POINT('Ctrl Pts',(-38.2872235270282,199.284874589309,-56.783650812819));
#41983=CARTESIAN_POINT('Ctrl Pts',(-38.4051782991123,199.196109721127,-55.));
#41984=CARTESIAN_POINT('',(-47.,199.531133844866,-55.));
#41985=CARTESIAN_POINT('Ctrl Pts',(-47.0000000000002,199.531133844866,-55.));
#41986=CARTESIAN_POINT('Ctrl Pts',(-42.5403232540606,199.346764066249,-55.));
#41987=CARTESIAN_POINT('Ctrl Pts',(-38.4051782991124,199.196109721127,-55.));
#41988=CARTESIAN_POINT('Ctrl Pts',(-47.,199.531133844866,-55.));
#41989=CARTESIAN_POINT('Ctrl Pts',(-47.9409191594096,199.570032865355,-55.));
#41990=CARTESIAN_POINT('Ctrl Pts',(-48.922029941875,199.602939608104,-54.8270184848835));
#41991=CARTESIAN_POINT('Ctrl Pts',(-50.9084746105678,199.65289333989,-54.073774081225));
#41992=CARTESIAN_POINT('Ctrl Pts',(-51.8888445983889,199.666147836552,-53.4248639005959));
#41993=CARTESIAN_POINT('Ctrl Pts',(-53.4248639005959,199.666147836552,-51.8888445983889));
#41994=CARTESIAN_POINT('Ctrl Pts',(-54.073774081225,199.65289333989,-50.9084746105678));
#41995=CARTESIAN_POINT('Ctrl Pts',(-54.8270184848835,199.602939608103,-48.922029941875));
#41996=CARTESIAN_POINT('Ctrl Pts',(-55.,199.570032865355,-47.9409191594096));
#41997=CARTESIAN_POINT('Ctrl Pts',(-55.,199.531133844866,-47.));
#41998=CARTESIAN_POINT('Origin',(0.,199.004037328772,-3.18971646165771E-15));
#41999=CARTESIAN_POINT('',(-47.,199.531133844866,55.));
#42000=CARTESIAN_POINT('Ctrl Pts',(-55.,199.531133844866,47.));
#42001=CARTESIAN_POINT('Ctrl Pts',(-55.,199.570032865355,47.9409191594096));
#42002=CARTESIAN_POINT('Ctrl Pts',(-54.8270184848835,199.602939608103,48.922029941875));
#42003=CARTESIAN_POINT('Ctrl Pts',(-54.073774081225,199.65289333989,50.9084746105678));
#42004=CARTESIAN_POINT('Ctrl Pts',(-53.4248639005959,199.666147836552,51.8888445983889));
#42005=CARTESIAN_POINT('Ctrl Pts',(-51.8888445983889,199.666147836552,53.4248639005959));
#42006=CARTESIAN_POINT('Ctrl Pts',(-50.9084746105678,199.65289333989,54.073774081225));
#42007=CARTESIAN_POINT('Ctrl Pts',(-48.922029941875,199.602939608103,54.8270184848835));
#42008=CARTESIAN_POINT('Ctrl Pts',(-47.9409191594096,199.570032865355,55.));
#42009=CARTESIAN_POINT('Ctrl Pts',(-47.,199.531133844866,55.));
#42010=CARTESIAN_POINT('',(-32.85003536606,199.004037328772,55.));
#42011=CARTESIAN_POINT('Ctrl Pts',(-32.85003536606,199.004037328772,55.));
#42012=CARTESIAN_POINT('Ctrl Pts',(-39.4954174846828,199.22088305859,55.));
#42013=CARTESIAN_POINT('Ctrl Pts',(-47.0000000000002,199.531133844866,55.));
#42014=CARTESIAN_POINT('',(32.8500353660599,199.004037328772,55.));
#42015=CARTESIAN_POINT('Origin',(-1.96137728289756E-15,199.004037328772,
0.));
#42016=CARTESIAN_POINT('',(47.,199.531133844866,55.));
#42017=CARTESIAN_POINT('Ctrl Pts',(47.0000000000002,199.531133844866,55.));
#42018=CARTESIAN_POINT('Ctrl Pts',(39.4954174846765,199.22088305859,55.));
#42019=CARTESIAN_POINT('Ctrl Pts',(32.8500353660488,199.004037328771,55.));
#42020=CARTESIAN_POINT('',(55.,199.531133844866,47.));
#42021=CARTESIAN_POINT('Ctrl Pts',(47.,199.531133844866,55.));
#42022=CARTESIAN_POINT('Ctrl Pts',(47.9409191594096,199.570032865355,55.));
#42023=CARTESIAN_POINT('Ctrl Pts',(48.922029941875,199.602939608104,54.8270184848835));
#42024=CARTESIAN_POINT('Ctrl Pts',(50.9084746105678,199.65289333989,54.073774081225));
#42025=CARTESIAN_POINT('Ctrl Pts',(51.8888445983889,199.666147836552,53.4248639005959));
#42026=CARTESIAN_POINT('Ctrl Pts',(53.4248639005959,199.666147836552,51.8888445983889));
#42027=CARTESIAN_POINT('Ctrl Pts',(54.073774081225,199.65289333989,50.9084746105678));
#42028=CARTESIAN_POINT('Ctrl Pts',(54.8270184848835,199.602939608103,48.922029941875));
#42029=CARTESIAN_POINT('Ctrl Pts',(55.,199.570032865355,47.9409191594096));
#42030=CARTESIAN_POINT('Ctrl Pts',(55.,199.531133844866,47.));
#42031=CARTESIAN_POINT('',(55.,199.004037328772,32.85003536606));
#42032=CARTESIAN_POINT('Ctrl Pts',(55.,199.004037328772,32.85003536606));
#42033=CARTESIAN_POINT('Ctrl Pts',(55.,199.22088305859,39.4954174846828));
#42034=CARTESIAN_POINT('Ctrl Pts',(55.,199.531133844866,47.0000000000002));
#42035=CARTESIAN_POINT('',(55.,199.004037328772,-32.85003536606));
#42036=CARTESIAN_POINT('Origin',(0.,199.004037328772,3.92275456579511E-15));
#42037=CARTESIAN_POINT('',(55.,199.531133844866,-47.));
#42038=CARTESIAN_POINT('Ctrl Pts',(55.,199.531133844866,-47.0000000000002));
#42039=CARTESIAN_POINT('Ctrl Pts',(55.,199.22088305859,-39.4954174846766));
#42040=CARTESIAN_POINT('Ctrl Pts',(55.,199.004037328771,-32.8500353660488));
#42041=CARTESIAN_POINT('',(47.,199.531133844866,-55.));
#42042=CARTESIAN_POINT('Ctrl Pts',(55.,199.531133844866,-47.));
#42043=CARTESIAN_POINT('Ctrl Pts',(55.,199.570032865355,-47.9409191594096));
#42044=CARTESIAN_POINT('Ctrl Pts',(54.8270184848835,199.602939608103,-48.922029941875));
#42045=CARTESIAN_POINT('Ctrl Pts',(54.073774081225,199.65289333989,-50.9084746105678));
#42046=CARTESIAN_POINT('Ctrl Pts',(53.4248639005959,199.666147836552,-51.8888445983889));
#42047=CARTESIAN_POINT('Ctrl Pts',(51.8888445983889,199.666147836552,-53.4248639005959));
#42048=CARTESIAN_POINT('Ctrl Pts',(50.9084746105678,199.65289333989,-54.073774081225));
#42049=CARTESIAN_POINT('Ctrl Pts',(48.922029941875,199.602939608103,-54.8270184848835));
#42050=CARTESIAN_POINT('Ctrl Pts',(47.9409191594096,199.570032865355,-55.));
#42051=CARTESIAN_POINT('Ctrl Pts',(47.,199.531133844866,-55.));
#42052=CARTESIAN_POINT('',(38.4051782991124,199.196109721127,-55.));
#42053=CARTESIAN_POINT('Ctrl Pts',(38.4051782991124,199.196109721127,-55.));
#42054=CARTESIAN_POINT('Ctrl Pts',(42.5403232540606,199.346764066249,-55.));
#42055=CARTESIAN_POINT('Ctrl Pts',(47.0000000000002,199.531133844866,-55.));
#42056=CARTESIAN_POINT('',(36.,200.,-71.1222000991162));
#42057=CARTESIAN_POINT('Ctrl Pts',(38.4051782991123,199.196109721126,-55.));
#42058=CARTESIAN_POINT('Ctrl Pts',(38.2872235270282,199.284874589309,-56.783650812819));
#42059=CARTESIAN_POINT('Ctrl Pts',(38.1547759803838,199.374640295943,-58.5623760439489));
#42060=CARTESIAN_POINT('Ctrl Pts',(37.8330351423798,199.560609339382,-62.2193907504964));
#42061=CARTESIAN_POINT('Ctrl Pts',(37.6420334379314,199.656620586686,-64.0895799742343));
#42062=CARTESIAN_POINT('Ctrl Pts',(37.2985629364648,199.784876737986,-66.6023010705813));
#42063=CARTESIAN_POINT('Ctrl Pts',(37.1771778906456,199.826039691768,-67.4102186809141));
#42064=CARTESIAN_POINT('Ctrl Pts',(36.9507101031668,199.886166180182,-68.608233824875));
#42065=CARTESIAN_POINT('Ctrl Pts',(36.8678693651456,199.905921405603,-69.0049790361478));
#42066=CARTESIAN_POINT('Ctrl Pts',(36.6773890334391,199.943421017973,-69.7728383598107));
#42067=CARTESIAN_POINT('Ctrl Pts',(36.5729453400847,199.961300812392,-70.1447351250176));
#42068=CARTESIAN_POINT('Ctrl Pts',(36.3559669090463,199.984858677538,-70.6735956916314));
#42069=CARTESIAN_POINT('Ctrl Pts',(36.2557708347516,199.994267844983,-70.8912518979424));
#42070=CARTESIAN_POINT('Ctrl Pts',(36.0894047422404,199.999088235995,-71.0608151548038));
#42071=CARTESIAN_POINT('Ctrl Pts',(36.0580820607069,199.999730794732,-71.088038844852));
#42072=CARTESIAN_POINT('Ctrl Pts',(36.0158673510785,199.999975166862,-71.1137294166545));
#42073=CARTESIAN_POINT('Ctrl Pts',(36.007998757625,200.,-71.1181513594252));
#42074=CARTESIAN_POINT('Ctrl Pts',(36.0000000000003,200.,-71.1222000991167));
#42075=CARTESIAN_POINT('Origin',(0.,200.,0.));
#42076=CARTESIAN_POINT('Origin',(0.,201.,0.));
#42077=CARTESIAN_POINT('',(55.,199.,32.6016382508379));
#42078=CARTESIAN_POINT('Ctrl Pts',(55.,199.,32.6016382508379));
#42079=CARTESIAN_POINT('Ctrl Pts',(55.,199.,32.6824692460632));
#42080=CARTESIAN_POINT('Ctrl Pts',(55.,199.001278753317,32.7654969801016));
#42081=CARTESIAN_POINT('Ctrl Pts',(55.,199.004037328772,32.85003536606));
#42082=CARTESIAN_POINT('',(55.,199.,-32.6016382508379));
#42083=CARTESIAN_POINT('Origin',(0.,199.,0.));
#42084=CARTESIAN_POINT('Ctrl Pts',(55.,199.004037328772,-32.85003536606));
#42085=CARTESIAN_POINT('Ctrl Pts',(55.,199.001278753317,-32.7654969801016));
#42086=CARTESIAN_POINT('Ctrl Pts',(55.,199.,-32.6824692460632));
#42087=CARTESIAN_POINT('Ctrl Pts',(55.,199.,-32.6016382508379));
#42088=CARTESIAN_POINT('Origin',(0.,199.,64.));
#42089=CARTESIAN_POINT('',(55.,199.,55.5));
#42090=CARTESIAN_POINT('Origin',(0.,201.,0.));
#42091=CARTESIAN_POINT('',(-32.6016382508379,199.,55.));
#42092=CARTESIAN_POINT('Ctrl Pts',(-32.6016382508379,199.,55.));
#42093=CARTESIAN_POINT('Ctrl Pts',(-32.6824692460632,199.,55.));
#42094=CARTESIAN_POINT('Ctrl Pts',(-32.7654969801016,199.001278753317,55.));
#42095=CARTESIAN_POINT('Ctrl Pts',(-32.85003536606,199.004037328772,55.));
#42096=CARTESIAN_POINT('',(32.6016382508379,199.,55.));
#42097=CARTESIAN_POINT('Origin',(0.,199.,0.));
#42098=CARTESIAN_POINT('Ctrl Pts',(32.8500353660599,199.004037328772,55.));
#42099=CARTESIAN_POINT('Ctrl Pts',(32.7654969801016,199.001278753317,55.));
#42100=CARTESIAN_POINT('Ctrl Pts',(32.6824692460632,199.,55.));
#42101=CARTESIAN_POINT('Ctrl Pts',(32.6016382508379,199.,55.));
#42102=CARTESIAN_POINT('Origin',(0.,199.,64.));
#42103=CARTESIAN_POINT('',(-23.5,199.,55.));
#42104=CARTESIAN_POINT('Origin',(0.,201.,0.));
#42105=CARTESIAN_POINT('Origin',(0.,199.,0.));
#42106=CARTESIAN_POINT('Origin',(0.,199.,64.));
#42107=CARTESIAN_POINT('Origin',(-73.,191.75,-138.));
#42108=CARTESIAN_POINT('',(-75.,201.,-138.));
#42109=CARTESIAN_POINT('Origin',(-73.,201.,-138.));
#42110=CARTESIAN_POINT('',(-75.,164.,-138.));
#42111=CARTESIAN_POINT('Origin',(-73.,164.,-138.));
#42112=CARTESIAN_POINT('',(-75.,191.75,-138.));
#42113=CARTESIAN_POINT('Ctrl Pts',(-73.,164.,-140.));
#42114=CARTESIAN_POINT('Ctrl Pts',(-73.,162.,-140.));
#42115=CARTESIAN_POINT('Ctrl Pts',(-71.,162.,-140.));
#42116=CARTESIAN_POINT('Ctrl Pts',(-75.,164.,-140.));
#42117=CARTESIAN_POINT('Ctrl Pts',(-75.,160.,-140.));
#42118=CARTESIAN_POINT('Ctrl Pts',(-71.,160.,-140.));
#42119=CARTESIAN_POINT('Ctrl Pts',(-75.,164.,-138.));
#42120=CARTESIAN_POINT('Ctrl Pts',(-75.,160.,-138.));
#42121=CARTESIAN_POINT('Ctrl Pts',(-71.,160.,-138.));
#42122=CARTESIAN_POINT('',(-71.,160.,-138.));
#42123=CARTESIAN_POINT('Origin',(-71.,162.,-138.));
#42124=CARTESIAN_POINT('Origin',(-71.,164.,-138.));
#42125=CARTESIAN_POINT('Origin',(-35.5,162.,-138.));
#42126=CARTESIAN_POINT('',(71.,160.,-138.));
#42127=CARTESIAN_POINT('Origin',(71.,162.,-138.));
#42128=CARTESIAN_POINT('',(-35.5,160.,-138.));
#42129=CARTESIAN_POINT('Ctrl Pts',(71.,162.,-140.));
#42130=CARTESIAN_POINT('Ctrl Pts',(73.,162.,-140.));
#42131=CARTESIAN_POINT('Ctrl Pts',(73.,164.,-140.));
#42132=CARTESIAN_POINT('Ctrl Pts',(71.,160.,-140.));
#42133=CARTESIAN_POINT('Ctrl Pts',(75.,160.,-140.));
#42134=CARTESIAN_POINT('Ctrl Pts',(75.,164.,-140.));
#42135=CARTESIAN_POINT('Ctrl Pts',(71.,160.,-138.));
#42136=CARTESIAN_POINT('Ctrl Pts',(75.,160.,-138.));
#42137=CARTESIAN_POINT('Ctrl Pts',(75.,164.,-138.));
#42138=CARTESIAN_POINT('',(75.,164.,-138.));
#42139=CARTESIAN_POINT('Origin',(73.,164.,-138.));
#42140=CARTESIAN_POINT('Origin',(71.,164.,-138.));
#42141=CARTESIAN_POINT('Origin',(73.,173.25,-138.));
#42142=CARTESIAN_POINT('',(75.,201.,-138.));
#42143=CARTESIAN_POINT('Origin',(73.,201.,-138.));
#42144=CARTESIAN_POINT('',(75.,173.25,-138.));
#42145=CARTESIAN_POINT('Ctrl Pts',(73.,201.,-140.));
#42146=CARTESIAN_POINT('Ctrl Pts',(73.,203.,-140.));
#42147=CARTESIAN_POINT('Ctrl Pts',(71.,203.,-140.));
#42148=CARTESIAN_POINT('Ctrl Pts',(75.,201.,-140.));
#42149=CARTESIAN_POINT('Ctrl Pts',(75.,205.,-140.));
#42150=CARTESIAN_POINT('Ctrl Pts',(71.,205.,-140.));
#42151=CARTESIAN_POINT('Ctrl Pts',(75.,201.,-138.));
#42152=CARTESIAN_POINT('Ctrl Pts',(75.,205.,-138.));
#42153=CARTESIAN_POINT('Ctrl Pts',(71.,205.,-138.));
#42154=CARTESIAN_POINT('',(71.,205.,-138.));
#42155=CARTESIAN_POINT('Origin',(71.,203.,-138.));
#42156=CARTESIAN_POINT('Origin',(71.,201.,-138.));
#42157=CARTESIAN_POINT('Origin',(35.5,203.,-138.));
#42158=CARTESIAN_POINT('',(-71.,205.,-138.));
#42159=CARTESIAN_POINT('Origin',(-71.,203.,-138.));
#42160=CARTESIAN_POINT('',(35.5,205.,-138.));
#42161=CARTESIAN_POINT('Ctrl Pts',(-71.,203.,-140.));
#42162=CARTESIAN_POINT('Ctrl Pts',(-73.,203.,-140.));
#42163=CARTESIAN_POINT('Ctrl Pts',(-73.,201.,-140.));
#42164=CARTESIAN_POINT('Ctrl Pts',(-71.,205.,-140.));
#42165=CARTESIAN_POINT('Ctrl Pts',(-75.,205.,-140.));
#42166=CARTESIAN_POINT('Ctrl Pts',(-75.,201.,-140.));
#42167=CARTESIAN_POINT('Ctrl Pts',(-71.,205.,-138.));
#42168=CARTESIAN_POINT('Ctrl Pts',(-75.,205.,-138.));
#42169=CARTESIAN_POINT('Ctrl Pts',(-75.,201.,-138.));
#42170=CARTESIAN_POINT('Origin',(-71.,201.,-138.));
#42171=CARTESIAN_POINT('Origin',(71.,201.,-140.));
#42172=CARTESIAN_POINT('',(71.,205.,-140.));
#42173=CARTESIAN_POINT('',(75.,201.,-140.));
#42174=CARTESIAN_POINT('Origin',(71.,205.,-140.));
#42175=CARTESIAN_POINT('',(-71.,205.,-140.));
#42176=CARTESIAN_POINT('Origin',(-71.,201.,-140.));
#42177=CARTESIAN_POINT('',(-75.,201.,-140.));
#42178=CARTESIAN_POINT('Origin',(-75.,201.,-140.));
#42179=CARTESIAN_POINT('',(-75.,164.,-140.));
#42180=CARTESIAN_POINT('Origin',(0.,213.,0.));
#42181=CARTESIAN_POINT('',(-1.53080849893419E-14,213.,-125.));
#42182=CARTESIAN_POINT('Origin',(-1.50631556295124E-14,213.,-123.));
#42183=CARTESIAN_POINT('Origin',(0.,213.,0.));
#42184=CARTESIAN_POINT('Origin',(0.,209.75,0.));
#42185=CARTESIAN_POINT('',(-1.53080849893419E-14,209.75,-125.));
#42186=CARTESIAN_POINT('',(0.,209.75,-125.));
#42187=CARTESIAN_POINT('Origin',(0.,205.,0.));
#42188=CARTESIAN_POINT('',(0.,203.,-47.));
#42189=CARTESIAN_POINT('Origin',(0.,203.,0.));
#42190=CARTESIAN_POINT('',(-5.51091059616309E-15,205.,-45.));
#42191=CARTESIAN_POINT('Origin',(-5.75583995599256E-15,205.,-47.));
#42192=CARTESIAN_POINT('Origin',(0.,205.,0.));
#42193=CARTESIAN_POINT('',(47.,203.,0.));
#42194=CARTESIAN_POINT('Origin',(0.,203.,0.));
#42195=CARTESIAN_POINT('',(0.,203.,47.));
#42196=CARTESIAN_POINT('Origin',(0.,203.,0.));
#42197=CARTESIAN_POINT('Origin',(0.,203.,0.));
#42198=CARTESIAN_POINT('Origin',(0.,203.,0.));
#42199=CARTESIAN_POINT('',(47.,203.,41.));
#42200=CARTESIAN_POINT('',(47.,203.,-41.));
#42201=CARTESIAN_POINT('',(41.,203.,47.));
#42202=CARTESIAN_POINT('Origin',(41.,203.,41.));
#42203=CARTESIAN_POINT('',(41.,203.,47.));
#42204=CARTESIAN_POINT('Origin',(0.,203.,0.));
#42205=CARTESIAN_POINT('',(41.,203.,-47.));
#42206=CARTESIAN_POINT('',(-41.,203.,-47.));
#42207=CARTESIAN_POINT('',(47.,203.,-41.));
#42208=CARTESIAN_POINT('Origin',(41.,203.,-41.));
#42209=CARTESIAN_POINT('',(47.,203.,-41.));
#42210=CARTESIAN_POINT('Origin',(0.,203.,0.));
#42211=CARTESIAN_POINT('',(-41.,203.,-47.));
#42212=CARTESIAN_POINT('Origin',(0.,203.,0.));
#42213=CARTESIAN_POINT('',(-41.,203.,47.));
#42214=CARTESIAN_POINT('',(41.,203.,47.));
#42215=CARTESIAN_POINT('Origin',(-41.,203.,41.));
#42216=CARTESIAN_POINT('Origin',(0.,207.,0.));
#42217=CARTESIAN_POINT('',(5.51091059616309E-15,209.,-45.));
#42218=CARTESIAN_POINT('Origin',(0.,209.,0.));
#42219=CARTESIAN_POINT('',(-5.51091059616309E-15,207.,-45.));
#42220=CARTESIAN_POINT('Origin',(0.,213.,0.));
#42221=CARTESIAN_POINT('',(-1.10340676603177E-14,213.,90.1));
#42222=CARTESIAN_POINT('Origin',(-1.12789970201471E-14,213.,92.1));
#42223=CARTESIAN_POINT('',(1.10340676603177E-14,213.,-90.1));
#42224=CARTESIAN_POINT('Origin',(0.,213.,0.));
#42225=CARTESIAN_POINT('Origin',(0.,213.,0.));
#42226=CARTESIAN_POINT('Origin',(0.,213.05,0.));
#42227=CARTESIAN_POINT('',(-1.10340676603177E-14,211.,-90.1));
#42228=CARTESIAN_POINT('Origin',(0.,211.,0.));
#42229=CARTESIAN_POINT('',(-1.10340676603177E-14,213.05,-90.1));
#42230=CARTESIAN_POINT('Origin',(0.,209.,0.));
#42231=CARTESIAN_POINT('',(-5.75583995599256E-15,211.,-47.));
#42232=CARTESIAN_POINT('Origin',(-5.75583995599256E-15,209.,-47.));
#42233=CARTESIAN_POINT('Origin',(0.,211.,0.));
#42234=CARTESIAN_POINT('Origin',(0.,211.,90.1));
#42235=CARTESIAN_POINT('Origin',(53.,139.,32.));
#42236=CARTESIAN_POINT('',(55.,148.,32.));
#42237=CARTESIAN_POINT('',(53.,148.,30.));
#42238=CARTESIAN_POINT('Origin',(53.,148.,32.));
#42239=CARTESIAN_POINT('',(53.,186.,30.));
#42240=CARTESIAN_POINT('',(53.,139.,30.));
#42241=CARTESIAN_POINT('',(55.,186.,32.));
#42242=CARTESIAN_POINT('Origin',(53.,186.,32.));
#42243=CARTESIAN_POINT('',(55.,139.,32.));
#42244=CARTESIAN_POINT('Origin',(53.,186.,24.));
#42245=CARTESIAN_POINT('',(53.,192.,24.));
#42246=CARTESIAN_POINT('',(55.,194.,24.));
#42247=CARTESIAN_POINT('Origin',(53.,194.,24.));
#42248=CARTESIAN_POINT('Origin',(55.,186.,24.));
#42249=CARTESIAN_POINT('Origin',(53.,186.,24.));
#42250=CARTESIAN_POINT('Origin',(53.,194.,35.5));
#42251=CARTESIAN_POINT('',(53.,192.,-24.));
#42252=CARTESIAN_POINT('',(55.,194.,-24.));
#42253=CARTESIAN_POINT('Origin',(53.,194.,-24.));
#42254=CARTESIAN_POINT('',(55.,194.,35.5));
#42255=CARTESIAN_POINT('',(53.,192.,35.5));
#42256=CARTESIAN_POINT('Origin',(53.,186.,-24.));
#42257=CARTESIAN_POINT('',(53.,186.,-30.));
#42258=CARTESIAN_POINT('',(55.,186.,-32.));
#42259=CARTESIAN_POINT('Origin',(53.,186.,-32.));
#42260=CARTESIAN_POINT('Origin',(55.,186.,-24.));
#42261=CARTESIAN_POINT('Origin',(53.,186.,-24.));
#42262=CARTESIAN_POINT('Origin',(53.,158.,-32.));
#42263=CARTESIAN_POINT('',(53.,148.,-30.));
#42264=CARTESIAN_POINT('',(55.,148.,-32.));
#42265=CARTESIAN_POINT('Origin',(53.,148.,-32.));
#42266=CARTESIAN_POINT('',(55.,158.,-32.));
#42267=CARTESIAN_POINT('',(53.,158.,-30.));
#42268=CARTESIAN_POINT('Origin',(53.,148.,-24.));
#42269=CARTESIAN_POINT('',(53.,142.,-24.));
#42270=CARTESIAN_POINT('',(55.,140.,-24.));
#42271=CARTESIAN_POINT('Origin',(53.,140.,-24.));
#42272=CARTESIAN_POINT('Origin',(55.,148.,-24.));
#42273=CARTESIAN_POINT('Origin',(53.,148.,-24.));
#42274=CARTESIAN_POINT('Origin',(53.,140.,11.5));
#42275=CARTESIAN_POINT('',(53.,142.,24.));
#42276=CARTESIAN_POINT('',(55.,140.,24.));
#42277=CARTESIAN_POINT('Origin',(53.,140.,24.));
#42278=CARTESIAN_POINT('',(55.,140.,11.5));
#42279=CARTESIAN_POINT('',(53.,142.,11.5));
#42280=CARTESIAN_POINT('Origin',(53.,148.,24.));
#42281=CARTESIAN_POINT('Origin',(55.,148.,24.));
#42282=CARTESIAN_POINT('Origin',(53.,148.,24.));
#42283=CARTESIAN_POINT('Origin',(55.,186.,-24.));
#42284=CARTESIAN_POINT('',(49.,192.,-24.));
#42285=CARTESIAN_POINT('',(55.,192.,-24.));
#42286=CARTESIAN_POINT('',(49.,186.,-30.));
#42287=CARTESIAN_POINT('Origin',(49.,186.,-24.));
#42288=CARTESIAN_POINT('',(55.,186.,-30.));
#42289=CARTESIAN_POINT('Origin',(55.,192.,24.));
#42290=CARTESIAN_POINT('',(49.,192.,24.));
#42291=CARTESIAN_POINT('',(55.,192.,24.));
#42292=CARTESIAN_POINT('',(49.,192.,32.5));
#42293=CARTESIAN_POINT('Origin',(55.,186.,24.));
#42294=CARTESIAN_POINT('',(49.,186.,30.));
#42295=CARTESIAN_POINT('',(55.,186.,30.));
#42296=CARTESIAN_POINT('Origin',(49.,186.,24.));
#42297=CARTESIAN_POINT('Origin',(55.,148.,30.));
#42298=CARTESIAN_POINT('',(49.,148.,30.));
#42299=CARTESIAN_POINT('',(55.,148.,30.));
#42300=CARTESIAN_POINT('',(49.,141.,30.));
#42301=CARTESIAN_POINT('Origin',(55.,130.,47.));
#42302=CARTESIAN_POINT('',(55.,132.,-47.));
#42303=CARTESIAN_POINT('',(55.,132.,47.));
#42304=CARTESIAN_POINT('',(55.,132.,23.5));
#42305=CARTESIAN_POINT('',(55.,130.,-47.));
#42306=CARTESIAN_POINT('',(55.,130.,47.));
#42307=CARTESIAN_POINT('Origin',(49.,141.,32.));
#42308=CARTESIAN_POINT('',(47.,186.,32.));
#42309=CARTESIAN_POINT('Origin',(49.,186.,32.));
#42310=CARTESIAN_POINT('',(47.,148.,32.));
#42311=CARTESIAN_POINT('Origin',(49.,148.,32.));
#42312=CARTESIAN_POINT('',(47.,141.,32.));
#42313=CARTESIAN_POINT('Origin',(49.,148.,24.));
#42314=CARTESIAN_POINT('',(49.,142.,24.));
#42315=CARTESIAN_POINT('',(47.,140.,24.));
#42316=CARTESIAN_POINT('Origin',(49.,140.,24.));
#42317=CARTESIAN_POINT('Origin',(47.,148.,24.));
#42318=CARTESIAN_POINT('Origin',(49.,148.,24.));
#42319=CARTESIAN_POINT('Origin',(49.,140.,8.5));
#42320=CARTESIAN_POINT('',(49.,142.,-24.));
#42321=CARTESIAN_POINT('',(47.,140.,-24.));
#42322=CARTESIAN_POINT('Origin',(49.,140.,-24.));
#42323=CARTESIAN_POINT('',(47.,140.,8.5));
#42324=CARTESIAN_POINT('',(49.,142.,8.5));
#42325=CARTESIAN_POINT('Origin',(49.,148.,-24.));
#42326=CARTESIAN_POINT('',(49.,148.,-30.));
#42327=CARTESIAN_POINT('',(47.,148.,-32.));
#42328=CARTESIAN_POINT('Origin',(49.,148.,-32.));
#42329=CARTESIAN_POINT('Origin',(47.,148.,-24.));
#42330=CARTESIAN_POINT('Origin',(49.,148.,-24.));
#42331=CARTESIAN_POINT('Origin',(49.,160.,-32.));
#42332=CARTESIAN_POINT('',(47.,186.,-32.));
#42333=CARTESIAN_POINT('Origin',(49.,186.,-32.));
#42334=CARTESIAN_POINT('',(47.,160.,-32.));
#42335=CARTESIAN_POINT('',(49.,160.,-30.));
#42336=CARTESIAN_POINT('Origin',(49.,186.,-24.));
#42337=CARTESIAN_POINT('',(47.,194.,-24.));
#42338=CARTESIAN_POINT('Origin',(49.,194.,-24.));
#42339=CARTESIAN_POINT('Origin',(47.,186.,-24.));
#42340=CARTESIAN_POINT('Origin',(49.,194.,32.5));
#42341=CARTESIAN_POINT('',(47.,194.,24.));
#42342=CARTESIAN_POINT('Origin',(49.,194.,24.));
#42343=CARTESIAN_POINT('',(47.,194.,32.5));
#42344=CARTESIAN_POINT('Origin',(49.,186.,24.));
#42345=CARTESIAN_POINT('Origin',(47.,186.,24.));
#42346=CARTESIAN_POINT('Origin',(55.,148.,-24.));
#42347=CARTESIAN_POINT('',(55.,148.,-30.));
#42348=CARTESIAN_POINT('',(55.,142.,-24.));
#42349=CARTESIAN_POINT('Origin',(55.,142.,-24.));
#42350=CARTESIAN_POINT('',(55.,142.,24.));
#42351=CARTESIAN_POINT('Origin',(55.,148.,24.));
#42352=CARTESIAN_POINT('Origin',(47.,134.,41.));
#42353=CARTESIAN_POINT('',(47.,134.,41.));
#42354=CARTESIAN_POINT('',(47.,134.,-41.));
#42355=CARTESIAN_POINT('Origin',(-53.,132.,-23.5));
#42356=CARTESIAN_POINT('',(-53.,130.,47.));
#42357=CARTESIAN_POINT('Origin',(-53.,132.,47.));
#42358=CARTESIAN_POINT('',(-53.,130.,-47.));
#42359=CARTESIAN_POINT('Origin',(-53.,132.,-47.));
#42360=CARTESIAN_POINT('',(-53.,130.,-23.5));
#42361=CARTESIAN_POINT('Origin',(-47.,132.,-47.));
#42362=CARTESIAN_POINT('',(-47.,132.,-55.));
#42363=CARTESIAN_POINT('',(-47.,130.,-53.));
#42364=CARTESIAN_POINT('Origin',(-47.,132.,-53.));
#42365=CARTESIAN_POINT('Origin',(-47.,130.,-47.));
#42366=CARTESIAN_POINT('Origin',(-47.,132.,-47.));
#42367=CARTESIAN_POINT('Origin',(23.5,132.,-53.));
#42368=CARTESIAN_POINT('',(47.,132.,-55.));
#42369=CARTESIAN_POINT('',(47.,130.,-53.));
#42370=CARTESIAN_POINT('Origin',(47.,132.,-53.));
#42371=CARTESIAN_POINT('',(23.5,130.,-53.));
#42372=CARTESIAN_POINT('',(23.5,132.,-55.));
#42373=CARTESIAN_POINT('Origin',(47.,132.,-47.));
#42374=CARTESIAN_POINT('',(53.,130.,-47.));
#42375=CARTESIAN_POINT('Origin',(53.,132.,-47.));
#42376=CARTESIAN_POINT('Origin',(47.,130.,-47.));
#42377=CARTESIAN_POINT('Origin',(47.,132.,-47.));
#42378=CARTESIAN_POINT('Origin',(53.,132.,23.5));
#42379=CARTESIAN_POINT('',(53.,130.,47.));
#42380=CARTESIAN_POINT('Origin',(53.,132.,47.));
#42381=CARTESIAN_POINT('',(53.,130.,23.5));
#42382=CARTESIAN_POINT('Origin',(47.,132.,47.));
#42383=CARTESIAN_POINT('',(47.,132.,55.));
#42384=CARTESIAN_POINT('',(47.,130.,53.));
#42385=CARTESIAN_POINT('Origin',(47.,132.,53.));
#42386=CARTESIAN_POINT('Origin',(47.,130.,47.));
#42387=CARTESIAN_POINT('Origin',(47.,132.,47.));
#42388=CARTESIAN_POINT('Origin',(-23.5,132.,53.));
#42389=CARTESIAN_POINT('',(-47.,132.,55.));
#42390=CARTESIAN_POINT('',(-47.,130.,53.));
#42391=CARTESIAN_POINT('Origin',(-47.,132.,53.));
#42392=CARTESIAN_POINT('',(-23.5,130.,53.));
#42393=CARTESIAN_POINT('',(-23.5,132.,55.));
#42394=CARTESIAN_POINT('Origin',(-47.,132.,47.));
#42395=CARTESIAN_POINT('Origin',(-47.,132.,47.));
#42396=CARTESIAN_POINT('Origin',(-47.,130.,47.));
#42397=CARTESIAN_POINT('Origin',(47.,130.,-47.));
#42398=CARTESIAN_POINT('',(47.,130.,-55.));
#42399=CARTESIAN_POINT('Origin',(47.,130.,-55.));
#42400=CARTESIAN_POINT('',(-47.,130.,-55.));
#42401=CARTESIAN_POINT('',(-40.,196.,-55.));
#42402=CARTESIAN_POINT('Origin',(-36.,196.,-55.));
#42403=CARTESIAN_POINT('',(-40.,169.,-55.));
#42404=CARTESIAN_POINT('',(-40.,163.,-55.));
#42405=CARTESIAN_POINT('',(-36.,165.,-55.));
#42406=CARTESIAN_POINT('Origin',(-36.,169.,-55.));
#42407=CARTESIAN_POINT('',(36.,165.,-55.));
#42408=CARTESIAN_POINT('',(5.5,165.,-55.));
#42409=CARTESIAN_POINT('',(40.,169.,-55.));
#42410=CARTESIAN_POINT('Origin',(36.,169.,-55.));
#42411=CARTESIAN_POINT('',(40.,196.,-55.));
#42412=CARTESIAN_POINT('',(40.,149.5,-55.));
#42413=CARTESIAN_POINT('Origin',(36.,196.,-55.));
#42414=CARTESIAN_POINT('Origin',(-47.,130.,-47.));
#42415=CARTESIAN_POINT('Origin',(0.,130.,0.));
#42416=CARTESIAN_POINT('',(4.9326051632324E-15,130.,-40.2777777777778));
#42417=CARTESIAN_POINT('Origin',(0.,130.,0.));
#42418=CARTESIAN_POINT('Origin',(-53.,194.,-35.5));
#42419=CARTESIAN_POINT('',(-53.,192.,-24.));
#42420=CARTESIAN_POINT('Origin',(-53.,194.,-24.));
#42421=CARTESIAN_POINT('',(-53.,192.,24.));
#42422=CARTESIAN_POINT('',(-53.,192.,-35.5));
#42423=CARTESIAN_POINT('Origin',(-53.,194.,24.));
#42424=CARTESIAN_POINT('Origin',(-53.,186.,24.));
#42425=CARTESIAN_POINT('',(-53.,186.,30.));
#42426=CARTESIAN_POINT('Origin',(-53.,186.,32.));
#42427=CARTESIAN_POINT('Origin',(-53.,186.,24.));
#42428=CARTESIAN_POINT('Origin',(-53.,158.,32.));
#42429=CARTESIAN_POINT('',(-53.,148.,30.));
#42430=CARTESIAN_POINT('Origin',(-53.,148.,32.));
#42431=CARTESIAN_POINT('',(-53.,158.,30.));
#42432=CARTESIAN_POINT('Origin',(-53.,148.,24.));
#42433=CARTESIAN_POINT('',(-53.,142.,24.));
#42434=CARTESIAN_POINT('Origin',(-53.,140.,24.));
#42435=CARTESIAN_POINT('Origin',(-53.,148.,24.));
#42436=CARTESIAN_POINT('Origin',(-53.,140.,-11.5));
#42437=CARTESIAN_POINT('',(-53.,142.,-24.));
#42438=CARTESIAN_POINT('Origin',(-53.,140.,-24.));
#42439=CARTESIAN_POINT('',(-53.,142.,-11.5));
#42440=CARTESIAN_POINT('Origin',(-53.,148.,-24.));
#42441=CARTESIAN_POINT('',(-53.,148.,-30.));
#42442=CARTESIAN_POINT('Origin',(-53.,148.,-32.));
#42443=CARTESIAN_POINT('Origin',(-53.,148.,-24.));
#42444=CARTESIAN_POINT('Origin',(-53.,139.,-32.));
#42445=CARTESIAN_POINT('',(-53.,186.,-30.));
#42446=CARTESIAN_POINT('Origin',(-53.,186.,-32.));
#42447=CARTESIAN_POINT('',(-53.,139.,-30.));
#42448=CARTESIAN_POINT('Origin',(-53.,186.,-24.));
#42449=CARTESIAN_POINT('Origin',(-53.,186.,-24.));
#42450=CARTESIAN_POINT('Origin',(-55.,148.,24.));
#42451=CARTESIAN_POINT('',(-49.,148.,30.));
#42452=CARTESIAN_POINT('',(-55.,148.,30.));
#42453=CARTESIAN_POINT('',(-49.,142.,24.));
#42454=CARTESIAN_POINT('Origin',(-49.,148.,24.));
#42455=CARTESIAN_POINT('',(-55.,142.,24.));
#42456=CARTESIAN_POINT('Origin',(-55.,186.,30.));
#42457=CARTESIAN_POINT('',(-49.,186.,30.));
#42458=CARTESIAN_POINT('',(-55.,186.,30.));
#42459=CARTESIAN_POINT('',(-49.,160.,30.));
#42460=CARTESIAN_POINT('Origin',(-55.,186.,24.));
#42461=CARTESIAN_POINT('',(-49.,192.,24.));
#42462=CARTESIAN_POINT('',(-55.,192.,24.));
#42463=CARTESIAN_POINT('Origin',(-49.,186.,24.));
#42464=CARTESIAN_POINT('Origin',(-55.,192.,-24.));
#42465=CARTESIAN_POINT('',(-49.,192.,-24.));
#42466=CARTESIAN_POINT('',(-55.,192.,-24.));
#42467=CARTESIAN_POINT('',(-49.,192.,-32.5));
#42468=CARTESIAN_POINT('Origin',(-49.,194.,-32.5));
#42469=CARTESIAN_POINT('Origin',(-49.,194.,24.));
#42470=CARTESIAN_POINT('Origin',(-49.,194.,-24.));
#42471=CARTESIAN_POINT('Origin',(-49.,186.,-24.));
#42472=CARTESIAN_POINT('',(-49.,186.,-30.));
#42473=CARTESIAN_POINT('Origin',(-49.,186.,-32.));
#42474=CARTESIAN_POINT('Origin',(-49.,186.,-24.));
#42475=CARTESIAN_POINT('Origin',(-49.,141.,-32.));
#42476=CARTESIAN_POINT('',(-49.,148.,-30.));
#42477=CARTESIAN_POINT('Origin',(-49.,148.,-32.));
#42478=CARTESIAN_POINT('',(-49.,141.,-30.));
#42479=CARTESIAN_POINT('Origin',(-49.,148.,-24.));
#42480=CARTESIAN_POINT('',(-49.,142.,-24.));
#42481=CARTESIAN_POINT('Origin',(-49.,140.,-24.));
#42482=CARTESIAN_POINT('Origin',(-49.,148.,-24.));
#42483=CARTESIAN_POINT('Origin',(-49.,140.,-8.5));
#42484=CARTESIAN_POINT('Origin',(-49.,140.,24.));
#42485=CARTESIAN_POINT('',(-49.,142.,-8.5));
#42486=CARTESIAN_POINT('Origin',(-49.,148.,24.));
#42487=CARTESIAN_POINT('Origin',(-49.,148.,32.));
#42488=CARTESIAN_POINT('Origin',(-49.,160.,32.));
#42489=CARTESIAN_POINT('Origin',(-49.,186.,32.));
#42490=CARTESIAN_POINT('Origin',(-49.,186.,24.));
#42491=CARTESIAN_POINT('Origin',(-55.,148.,-24.));
#42492=CARTESIAN_POINT('',(-55.,142.,-24.));
#42493=CARTESIAN_POINT('',(-55.,148.,-30.));
#42494=CARTESIAN_POINT('Origin',(-55.,148.,-30.));
#42495=CARTESIAN_POINT('',(-55.,186.,-30.));
#42496=CARTESIAN_POINT('Origin',(-55.,186.,-24.));
#42497=CARTESIAN_POINT('Origin',(-76.0139789775539,202.9,-76.0139789775538));
#42498=CARTESIAN_POINT('Origin',(-76.0139789775538,202.9,76.0139789775539));
#42499=CARTESIAN_POINT('Origin',(76.0139789775539,202.9,76.0139789775539));
#42500=CARTESIAN_POINT('Origin',(76.0139789775538,202.9,-76.0139789775539));
#42501=CARTESIAN_POINT('Origin',(-41.0121933088198,62.1,-41.0121933088198));
#42502=CARTESIAN_POINT('',(-46.5121933088198,62.1,-41.0121933088198));
#42503=CARTESIAN_POINT('Origin',(-41.0121933088198,62.1,41.0121933088198));
#42504=CARTESIAN_POINT('',(-46.5121933088198,62.1,41.0121933088198));
#42505=CARTESIAN_POINT('Origin',(41.0121933088198,62.1,41.0121933088198));
#42506=CARTESIAN_POINT('',(35.5121933088198,62.1,41.0121933088198));
#42507=CARTESIAN_POINT('Origin',(41.0121933088197,62.1,-41.0121933088198));
#42508=CARTESIAN_POINT('',(35.5121933088197,62.1,-41.0121933088198));
#42509=CARTESIAN_POINT('Origin',(-55.,142.,24.));
#42510=CARTESIAN_POINT('Origin',(55.,186.,-30.));
#42511=CARTESIAN_POINT('Origin',(0.,128.,27.5));
#42512=CARTESIAN_POINT('',(-3.36777869765522E-15,128.,-27.5));
#42513=CARTESIAN_POINT('Origin',(0.,128.,0.));
#42514=CARTESIAN_POINT('',(-3.18530632458227E-15,128.,-26.01));
#42515=CARTESIAN_POINT('Origin',(0.,128.,0.));
#42516=CARTESIAN_POINT('Origin',(0.,129.075,0.));
#42517=CARTESIAN_POINT('',(-3.36777869765522E-15,129.075,-27.5));
#42518=CARTESIAN_POINT('Origin',(0.,66.,26.01));
#42519=CARTESIAN_POINT('',(-3.18530632458227E-15,66.,-26.01));
#42520=CARTESIAN_POINT('Origin',(0.,66.,0.));
#42521=CARTESIAN_POINT('',(-2.75545529808154E-15,66.,-22.5));
#42522=CARTESIAN_POINT('Origin',(0.,66.,0.));
#42523=CARTESIAN_POINT('Origin',(0.,100.05,0.));
#42524=CARTESIAN_POINT('',(-3.18530632458227E-15,100.05,-26.01));
#42525=CARTESIAN_POINT('Origin',(41.,134.,41.));
#42526=CARTESIAN_POINT('',(41.,134.,47.));
#42527=CARTESIAN_POINT('Origin',(-41.,134.,47.));
#42528=CARTESIAN_POINT('',(-41.,134.,47.));
#42529=CARTESIAN_POINT('Origin',(-41.,134.,41.));
#42530=CARTESIAN_POINT('Origin',(41.,134.,-47.));
#42531=CARTESIAN_POINT('',(41.,134.,-47.));
#42532=CARTESIAN_POINT('Origin',(41.,134.,-41.));
#42533=CARTESIAN_POINT('Origin',(75.,164.,-140.));
#42534=CARTESIAN_POINT('',(75.,164.,-140.));
#42535=CARTESIAN_POINT('Origin',(71.,164.,-140.));
#42536=CARTESIAN_POINT('',(71.,160.,-140.));
#42537=CARTESIAN_POINT('Origin',(-71.,160.,-140.));
#42538=CARTESIAN_POINT('',(-71.,160.,-140.));
#42539=CARTESIAN_POINT('Origin',(-71.,164.,-140.));
#42540=CARTESIAN_POINT('Origin',(-36.,165.,-125.));
#42541=CARTESIAN_POINT('',(-36.,165.,-125.));
#42542=CARTESIAN_POINT('',(36.,165.,-125.));
#42543=CARTESIAN_POINT('Origin',(-36.,169.,-125.));
#42544=CARTESIAN_POINT('',(-40.,169.,-125.));
#42545=CARTESIAN_POINT('Origin',(-40.,196.,-125.));
#42546=CARTESIAN_POINT('',(-40.,196.,-125.));
#42547=CARTESIAN_POINT('Origin',(-36.,196.,-125.));
#42548=CARTESIAN_POINT('',(-36.,200.,-125.));
#42549=CARTESIAN_POINT('Origin',(36.,200.,-125.));
#42550=CARTESIAN_POINT('',(36.,200.,-125.));
#42551=CARTESIAN_POINT('Origin',(36.,196.,-125.));
#42552=CARTESIAN_POINT('',(40.,196.,-125.));
#42553=CARTESIAN_POINT('Origin',(40.,169.,-125.));
#42554=CARTESIAN_POINT('',(40.,169.,-125.));
#42555=CARTESIAN_POINT('Origin',(36.,169.,-125.));
#42556=CARTESIAN_POINT('Origin',(-47.,130.,55.));
#42557=CARTESIAN_POINT('',(47.,130.,55.));
#42558=CARTESIAN_POINT('',(-47.,130.,55.));
#42559=CARTESIAN_POINT('Origin',(-47.,130.,47.));
#42560=CARTESIAN_POINT('Origin',(47.,130.,47.));
#42561=CARTESIAN_POINT('Origin',(0.,91.,0.));
#42562=CARTESIAN_POINT('',(-2.75545529808154E-15,91.,-22.5));
#42563=CARTESIAN_POINT('Origin',(0.,98.,0.));
#42564=CARTESIAN_POINT('',(-5.20474889637625E-15,98.,-42.5));
#55697=UNCERTAINTY_MEASURE_WITH_UNIT(LENGTH_MEASURE(0.01),#55738,
'DISTANCE_ACCURACY_VALUE',
'Maximum model space distance between geometric entities at asserted c
onnectivities');
#55715=UNCERTAINTY_MEASURE_WITH_UNIT(LENGTH_MEASURE(0.01),#55738,
'DISTANCE_ACCURACY_VALUE',
'Maximum model space distance between geometric entities at asserted c
onnectivities');
#55719=(
GEOMETRIC_REPRESENTATION_CONTEXT(3)
GLOBAL_UNCERTAINTY_ASSIGNED_CONTEXT((#55697))
GLOBAL_UNIT_ASSIGNED_CONTEXT((#55738,#55740,#55741))
REPRESENTATION_CONTEXT('','3D')
);
#55737=(
GEOMETRIC_REPRESENTATION_CONTEXT(3)
GLOBAL_UNCERTAINTY_ASSIGNED_CONTEXT((#55715))
GLOBAL_UNIT_ASSIGNED_CONTEXT((#55738,#55740,#55741))
REPRESENTATION_CONTEXT('','3D')
);
#55738=(
LENGTH_UNIT()
NAMED_UNIT(*)
SI_UNIT(.MILLI.,.METRE.)
);
#55740=(
NAMED_UNIT(*)
PLANE_ANGLE_UNIT()
SI_UNIT($,.RADIAN.)
);
#55741=(
NAMED_UNIT(*)
SI_UNIT($,.STERADIAN.)
SOLID_ANGLE_UNIT()
);
#55745=SHAPE_DEFINITION_REPRESENTATION(#55766,#55823);
#55766=PRODUCT_DEFINITION_SHAPE('',$,#55845);
#55823=SHAPE_REPRESENTATION('',(#27989),#55719);
#55841=PRODUCT_DEFINITION_CONTEXT('part definition',#55906,'design');
#55845=PRODUCT_DEFINITION('2026-10-26-00-34-02-758',
'03_Bearing_Bracket_Motor_Adaptor',#55866,#55841);
#55866=PRODUCT_DEFINITION_FORMATION('',$,#55911);
#55906=APPLICATION_CONTEXT(
'Core Data for Automotive Mechanical Design Process');
#55907=PRODUCT_CONTEXT('part definition',#55906,'mechanical');
#55911=PRODUCT('2026-10-26-00-34-02-758',
'03_Bearing_Bracket_Motor_Adaptor',$,(#55907));
#55985=COLOUR_RGB('Grey',0.48,0.52,0.57);
#55986=FILL_AREA_STYLE_COLOUR('',#55985);
#55987=FILL_AREA_STYLE('',(#55986));
#55988=SURFACE_STYLE_FILL_AREA(#55987);
#55989=SURFACE_SIDE_STYLE('',(#55988));
#55990=SURFACE_STYLE_USAGE(.BOTH.,#55989);
#55991=PRESENTATION_STYLE_ASSIGNMENT((#55990));
ENDSEC;
END-ISO-10303-21;
